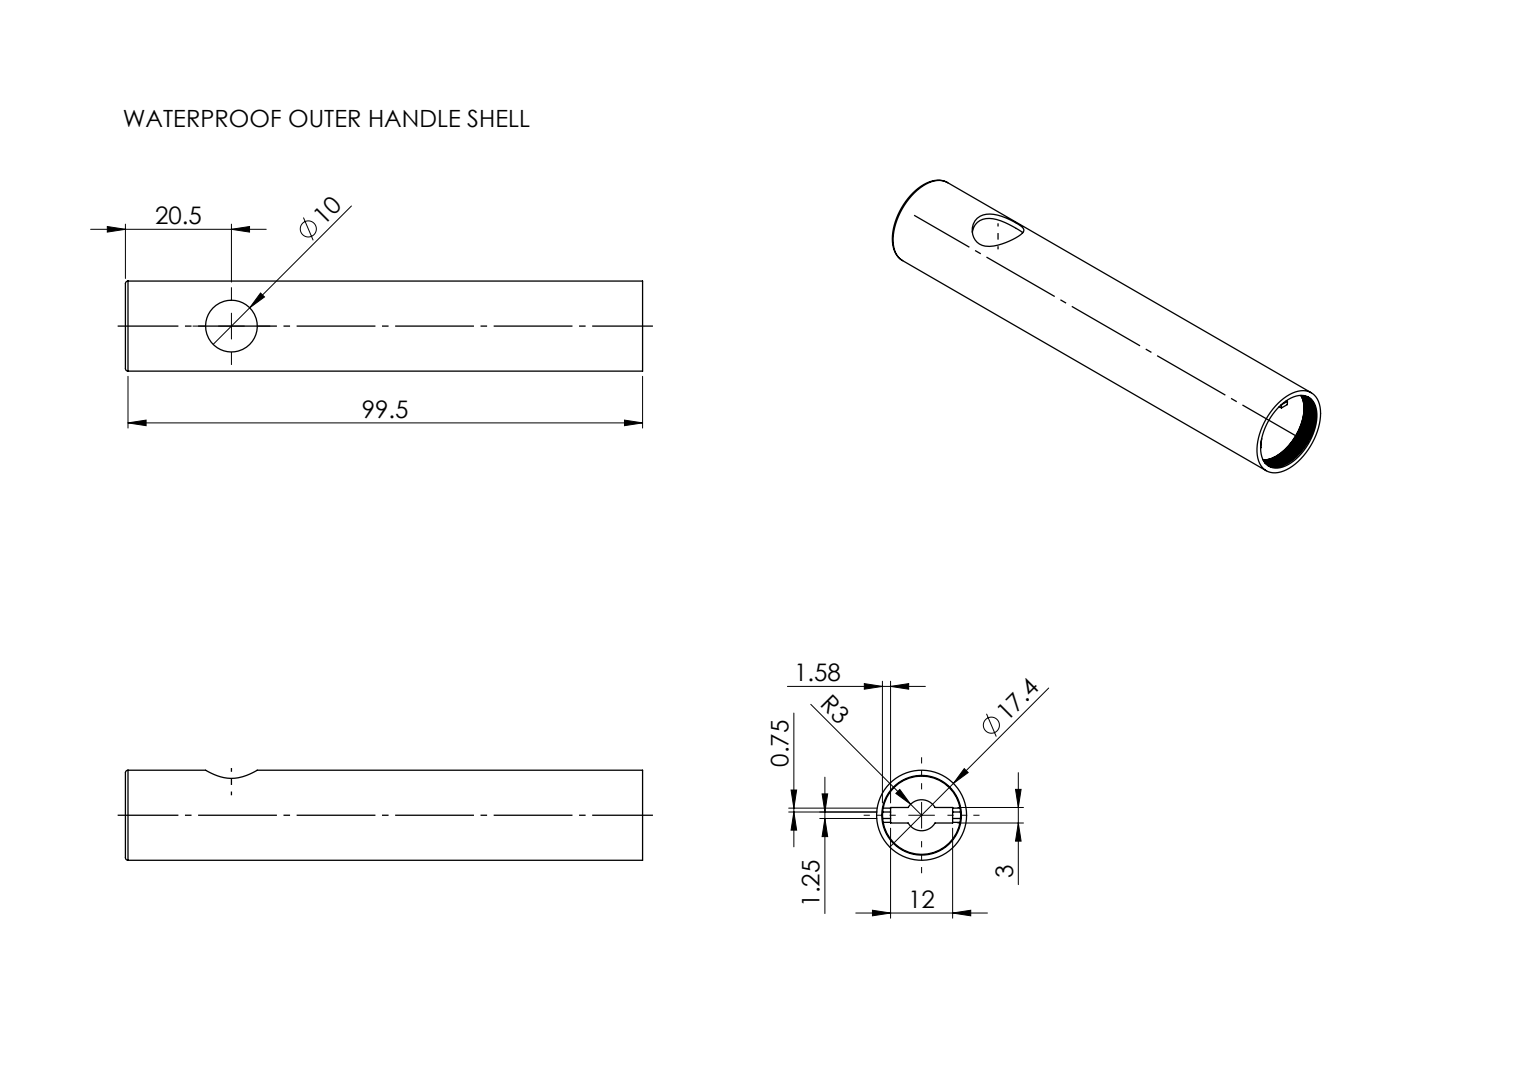
ISO-10303-21;
HEADER;
FILE_DESCRIPTION (('STEP AP214'),
    '1' );
FILE_NAME ('Waterproof Outer Handle Shell.step',
    '2026-10-02T09:26:43',
    ( '' ),
    ( '' ),
    'SwSTEP 2.0',
    'SolidWorks 2026',
    '' );
FILE_SCHEMA (( 'AUTOMOTIVE_DESIGN' ));
ENDSEC;

DATA;
#5=DIRECTION ( 'NONE',  ( -1.000000000000000000, -0.000000000000000000, -0.000000000000000000 ) ) ;
#32=DIRECTION ( 'NONE',  ( 0.000000000000000000, 0.000000000000000000, -1.000000000000000000 ) ) ;
#92=( BOUNDED_CURVE ( )  B_SPLINE_CURVE ( 2, ( #80530, #51076, #39332, #70696, #90980, #28848, #108684 ),
 .UNSPECIFIED., .F., .F. ) 
 B_SPLINE_CURVE_WITH_KNOTS ( ( 3, 2, 2, 3 ),
 ( 0.7142857142857148567, 0.7380952380952386926, 0.7619047619047624176, 0.7857142857142862535 ),
 .UNSPECIFIED. ) 
 CURVE ( )  GEOMETRIC_REPRESENTATION_ITEM ( )  RATIONAL_B_SPLINE_CURVE ( ( 0.9999999999999968914, 0.8660254037844418162, 1.000000000000000000, 0.8660254037844387076, 1.000000000000000000, 0.8660254037844355990, 1.000000000000003109 ) ) 
 REPRESENTATION_ITEM ( '' )  );
#144=CARTESIAN_POINT ( 'NONE',  ( 187.0677083336747160, -4.367472073101514418, -7.564683531250002702 ) ) ;
#216=ORIENTED_EDGE ( 'NONE', *, *, #25647, .T. ) ;
#223=EDGE_CURVE ( 'NONE', #51195, #50358, #69379, .T. ) ;
#245=EDGE_CURVE ( 'NONE', #43167, #39233, #13868, .T. ) ;
#256=CARTESIAN_POINT ( 'NONE',  ( 186.4218750003414016, 0.000000000000000000, 7.564683531250000925 ) ) ;
#346=CARTESIAN_POINT ( 'NONE',  ( 184.9427083336747160, -6.551208109652278289, 3.782341765624995134 ) ) ;
#354=CARTESIAN_POINT ( 'NONE',  ( 185.5000000000000000, 0.000000000000000000, 7.700000000000000178 ) ) ;
#507=CARTESIAN_POINT ( 'NONE',  ( 108.8430433244084554, 5.913955341756470752, 4.931228954127792719 ) ) ;
#548=CARTESIAN_POINT ( 'NONE',  ( 186.6927083336747160, 6.551208109652275624, -3.782341765624998686 ) ) ;
#601=( GEOMETRIC_REPRESENTATION_CONTEXT ( 3 ) GLOBAL_UNCERTAINTY_ASSIGNED_CONTEXT ( ( #63820 ) ) GLOBAL_UNIT_ASSIGNED_CONTEXT ( ( #82675, #124525, #32940 ) ) REPRESENTATION_CONTEXT ( 'NONE', 'WORKASPACE' ) );
#603=EDGE_LOOP ( 'NONE', ( #56647, #48064, #112160, #118008 ) ) ;
#644=CARTESIAN_POINT ( 'NONE',  ( 186.5312500006828031, 9.429780353434619030E-16, -7.700000000000000178 ) ) ;
#695=CARTESIAN_POINT ( 'NONE',  ( 185.9583333333333144, 4.445597072760159030, 7.699999999999928235 ) ) ;
#805=CARTESIAN_POINT ( 'NONE',  ( 103.6746308345937422, 8.329113074144254725, -2.529173134518388544 ) ) ;
#871=( BOUNDED_CURVE ( )  B_SPLINE_CURVE ( 2, ( #122989, #65333, #24143, #44418, #5760, #82436, #64062, #74530, #103993, #54246, #62787, #122352, #72603, #114441, #14300, #84347, #124279, #24787, #64699, #104620, #14922, #13000, #92895, #54872, #98660, #115730, #8351, #126205, #117004, #47654, #97383, #18820, #27336, #35892, #108489, #98027, #46344, #118313, #127501, #26719, #106553, #75801, #26080, #58758, #86258, #87556, #37194, #65989, #16856, #16225, #45722, #48292, #68564, #85630, #37824, #125549, #105924, #58122, #56160, #28661, #36556, #96095, #6393, #56790, #78416, #28006, #76467, #67243, #77727, #116371, #86913, #107199, #77108, #66628, #117642, #96726, #7054, #47014, #67923, #38495, #126857, #17525, #107850, #57473, #7702 ),
 .UNSPECIFIED., .F., .F. ) 
 B_SPLINE_CURVE_WITH_KNOTS ( ( 3, 2, 2, 2, 2, 2, 2, 2, 2, 2, 2, 2, 2, 2, 2, 2, 2, 2, 2, 2, 2, 2, 2, 2, 2, 2, 2, 2, 2, 2, 2, 2, 2, 2, 2, 2, 2, 2, 2, 2, 2, 2, 3 ),
 ( 0.000000000000000000, 0.02380952380952380820, 0.04761904761904761640, 0.07142857142857142461, 0.09523809523809523281, 0.1190476190476190410, 0.1428571428571428492, 0.1666666666666666574, 0.1904761904761904656, 0.2142857142857142738, 0.2380952380952380820, 0.2619047619047619180, 0.2857142857142856984, 0.3095238095238095344, 0.3333333333333333148, 0.3571428571428571508, 0.3809523809523809312, 0.4047619047619047672, 0.4285714285714285476, 0.4523809523809523836, 0.4761904761904761640, 0.5000000000000000000, 0.5238095238095238360, 0.5476190476190476719, 0.5714285714285713969, 0.5952380952380952328, 0.6190476190476190688, 0.6428571428571429047, 0.6666666666666666297, 0.6904761904761904656, 0.7142857142857143016, 0.7380952380952381375, 0.7619047619047618625, 0.7857142857142856984, 0.8095238095238095344, 0.8333333333333333703, 0.8571428571428570953, 0.8809523809523809312, 0.9047619047619047672, 0.9285714285714286031, 0.9523809523809523281, 0.9761904761904761640, 1.000000000000000000 ),
 .UNSPECIFIED. ) 
 CURVE ( )  GEOMETRIC_REPRESENTATION_ITEM ( )  RATIONAL_B_SPLINE_CURVE ( ( 1.000000000000000000, 0.8660254037844387076, 1.000000000000000000, 0.8660254037844387076, 1.000000000000000000, 0.8660254037844387076, 1.000000000000000000, 0.8660254037844387076, 1.000000000000000000, 0.8660254037844387076, 1.000000000000000000, 0.8660254037844387076, 1.000000000000000000, 0.8660254037844387076, 1.000000000000000000, 0.8660254037844387076, 1.000000000000000000, 0.8660254037844387076, 1.000000000000000000, 0.8660254037844387076, 1.000000000000000000, 0.8660254037844387076, 1.000000000000000000, 0.8660254037844387076, 1.000000000000000000, 0.8660254037844387076, 1.000000000000000000, 0.8660254037844387076, 1.000000000000000000, 0.8660254037844387076, 1.000000000000000000, 0.8660254037844387076, 1.000000000000000000, 0.8660254037844387076, 1.000000000000000000, 0.8660254037844387076, 1.000000000000000000, 0.8660254037844387076, 1.000000000000000000, 0.8660254037844387076, 1.000000000000000000, 0.8660254037844387076, 1.000000000000000000, 0.8660254037844387076, 1.000000000000000000, 0.8660254037844387076, 1.000000000000000000, 0.8660254037844387076, 1.000000000000000000, 0.8660254037844387076, 1.000000000000000000, 0.8660254037844387076, 1.000000000000000000, 0.8660254037844387076, 1.000000000000000000, 0.8660254037844387076, 1.000000000000000000, 0.8660254037844387076, 1.000000000000000000, 0.8660254037844387076, 1.000000000000000000, 0.8660254037844387076, 1.000000000000000000, 0.8660254037844387076, 1.000000000000000000, 0.8660254037844387076, 1.000000000000000000, 0.8660254037844387076, 1.000000000000000000, 0.8660254037844387076, 1.000000000000000000, 0.8660254037844387076, 1.000000000000000000, 0.8660254037844387076, 1.000000000000000000, 0.8660254037844387076, 1.000000000000000000, 0.8660254037844387076, 1.000000000000000000, 0.8660254037844387076, 1.000000000000000000, 0.8660254037844387076, 1.000000000000000000, 0.8660254037844387076, 1.000000000000000000 ) ) 
 REPRESENTATION_ITEM ( '' )  );
#888=CARTESIAN_POINT ( 'NONE',  ( 111.9626685488627942, 8.146665828590855085, 3.066327037116900023 ) ) ;
#912=EDGE_CURVE ( 'NONE', #19872, #5682, #21151, .T. ) ;
#921=CARTESIAN_POINT ( 'NONE',  ( 184.2916666666666856, 4.445597072760049784, -7.700000000000123634 ) ) ;
#993=ORIENTED_EDGE ( 'NONE', *, *, #126584, .F. ) ;
#1000=VERTEX_POINT ( 'NONE', #9044 ) ;
#1007=CARTESIAN_POINT ( 'NONE',  ( 183.9843750003414016, -8.734944146203032389, -1.604583208406768146E-15 ) ) ;
#1008=PLANE ( 'NONE',  #81316 ) ;
#1098=ORIENTED_EDGE ( 'NONE', *, *, #72625, .T. ) ;
#1111=AXIS2_PLACEMENT_3D ( 'NONE', #4715, #13259, #63021 ) ;
#1117=CARTESIAN_POINT ( 'NONE',  ( 187.5000000000000000, 0.000000000000000000, 0.000000000000000000 ) ) ;
#1139=DIRECTION ( 'NONE',  ( 0.000000000000000000, 1.000000000000000000, 0.000000000000000000 ) ) ;
#1204=CARTESIAN_POINT ( 'NONE',  ( 184.8593750003413732, 0.000000000000000000, 7.564683531250000925 ) ) ;
#1226=ADVANCED_FACE ( 'NONE', ( #124820 ), #52852, .F. ) ;
#1327=DIRECTION ( 'NONE',  ( -1.000000000000000000, -0.000000000000000000, -0.000000000000000000 ) ) ;
#1392=VERTEX_POINT ( 'NONE', #77482 ) ;
#1410=CARTESIAN_POINT ( 'NONE',  ( 183.8906250003414016, 0.000000000000000000, 7.564683531250000925 ) ) ;
#1445=CARTESIAN_POINT ( 'NONE',  ( 186.1093750003413732, 9.264065473108010111E-16, -7.564683531250000925 ) ) ;
#1551=CARTESIAN_POINT ( 'NONE',  ( 187.1302083336747444, -4.367472073101514418, -7.564683531250002702 ) ) ;
#1629=EDGE_CURVE ( 'NONE', #101564, #44902, #5358, .T. ) ;
#1630=B_SPLINE_CURVE_WITH_KNOTS ( 'NONE', 3,
 ( #25452, #14975, #54922, #124969, #75216, #57521, #49000, #29997, #90167, #9042, #69914, #78465, #28706, #127544, #88911, #98707, #118358, #8396, #60112, #20165, #98075, #88229, #67964, #97429, #107895, #48336, #68611, #7755, #89547, #100021, #10342, #128193, #50275, #507, #108546, #49645, #128861, #129506 ),
 .UNSPECIFIED., .F., .F.,
 ( 4, 2, 2, 2, 2, 2, 2, 2, 2, 2, 2, 2, 2, 2, 2, 2, 2, 2, 4 ),
 ( 0.000000000000000000, 0.001007299096406573174, 0.002014598192813146348, 0.003021897289219719306, 0.004029196385626292697, 0.005036495482032866088, 0.006043794578439438611, 0.007051093674846012002, 0.008058392771252585393, 0.008562042319455872089, 0.009065691867659158784, 0.01007299096406573218, 0.01108029006047230557, 0.01208758915687887722, 0.01309488825328545061, 0.01410218734969202400, 0.01510948644609859740, 0.01561313599430188409, 0.01611678554250517079 ),
 .UNSPECIFIED. ) ;
#1698=EDGE_CURVE ( 'NONE', #109625, #1000, #112399, .T. ) ;
#1819=ADVANCED_FACE ( 'NONE', ( #89728 ), #48520, .F. ) ;
#1840=ORIENTED_EDGE ( 'NONE', *, *, #49030, .T. ) ;
#1841=CARTESIAN_POINT ( 'NONE',  ( 186.2968750003414584, 8.734944146203032389, 5.348610694689227483E-16 ) ) ;
#1861=CYLINDRICAL_SURFACE ( 'NONE', #39546, 7.700000000000000178 ) ;
#1865=CARTESIAN_POINT ( 'NONE',  ( 127.5000000000000000, 0.000000000000000000, 0.000000000000000000 ) ) ;
#1966=ORIENTED_EDGE ( 'NONE', *, *, #68617, .F. ) ;
#1967=CARTESIAN_POINT ( 'NONE',  ( 103.0694403040216400, 7.655046866769239955, 0.8471574321703054800 ) ) ;
#2046=VERTEX_POINT ( 'NONE', #63497 ) ;
#2074=FACE_OUTER_BOUND ( 'NONE', #73731, .T. ) ;
#2081=CARTESIAN_POINT ( 'NONE',  ( 184.7760416670080588, 6.551208109652274736, 3.782341765625001351 ) ) ;
#2171=VERTEX_POINT ( 'NONE', #83148 ) ;
#2265=ORIENTED_EDGE ( 'NONE', *, *, #128795, .F. ) ;
#2305=CARTESIAN_POINT ( 'NONE',  ( 187.5000000000000000, -1.500000000000000000, 6.000000000000000000 ) ) ;
#2347=ORIENTED_EDGE ( 'NONE', *, *, #100683, .T. ) ;
#2370=( BOUNDED_CURVE ( )  B_SPLINE_CURVE ( 2, ( #36862, #103671, #76781, #74847, #23816, #114754, #54535 ),
 .UNSPECIFIED., .F., .F. ) 
 B_SPLINE_CURVE_WITH_KNOTS ( ( 3, 2, 2, 3 ),
 ( 0.2142857142857144681, 0.2380952380952383041, 0.2619047619047621955, 0.2857142857142859760 ),
 .UNSPECIFIED. ) 
 CURVE ( )  GEOMETRIC_REPRESENTATION_ITEM ( )  RATIONAL_B_SPLINE_CURVE ( ( 0.9999999999999988898, 0.8660254037844397068, 1.000000000000000000, 0.8660254037844387076, 1.000000000000000000, 0.8660254037844371533, 1.000000000000001554 ) ) 
 REPRESENTATION_ITEM ( '' )  );
#2428=CARTESIAN_POINT ( 'NONE',  ( 185.9479166673494603, -6.668395609140176816, -3.850000000000003642 ) ) ;
#2475=CARTESIAN_POINT ( 'NONE',  ( 186.3802083336747444, 4.367472073101515306, 7.564683531250000925 ) ) ;
#2523=EDGE_CURVE ( 'NONE', #39233, #127679, #43323, .T. ) ;
#2635=CARTESIAN_POINT ( 'NONE',  ( 186.0312500006828031, 9.429780353434619030E-16, -7.700000000000000178 ) ) ;
#2688=CARTESIAN_POINT ( 'NONE',  ( 108.0000000000000142, 8.700999999999998735, -5.000000000000004441 ) ) ;
#2711=CIRCLE ( 'NONE', #46527, 7.700000000000000178 ) ;
#2729=CARTESIAN_POINT ( 'NONE',  ( 185.2760416670080588, 6.551208109652274736, 3.782341765625001351 ) ) ;
#2798=DIRECTION ( 'NONE',  ( -1.000000000000000000, -0.000000000000000000, -0.000000000000000000 ) ) ;
#2847=CARTESIAN_POINT ( 'NONE',  ( 185.6718750003414016, 9.264065473108010111E-16, -7.564683531250000925 ) ) ;
#2865=VECTOR ( 'NONE', #65208, 1000.000000000000000 ) ;
#2879=CARTESIAN_POINT ( 'NONE',  ( 129.5000000000000000, 0.6250000000000025535, -6.000000000000000888 ) ) ;
#2922=CARTESIAN_POINT ( 'NONE',  ( 127.5000000000000000, 0.000000000000000000, 0.000000000000000000 ) ) ;
#2955=CARTESIAN_POINT ( 'NONE',  ( 187.5000000000000000, 9.429780353434619030E-16, -7.700000000000000178 ) ) ;
#2977=PLANE ( 'NONE',  #102632 ) ;
#3027=CARTESIAN_POINT ( 'NONE',  ( 187.5000000000000000, 0.000000000000000000, 0.000000000000000000 ) ) ;
#3105=CARTESIAN_POINT ( 'NONE',  ( 186.1145833340161175, 6.668395609140177704, -3.849999999999998312 ) ) ;
#3151=CARTESIAN_POINT ( 'NONE',  ( 186.3385416670080872, 6.551208109652274736, 3.782341765625001351 ) ) ;
#3193=EDGE_CURVE ( 'NONE', #125237, #48297, #19068, .T. ) ;
#3379=DIRECTION ( 'NONE',  ( 0.000000000000000000, 0.000000000000000000, -1.000000000000000000 ) ) ;
#3381=CARTESIAN_POINT ( 'NONE',  ( 184.4843750003414016, -8.734944146203032389, -1.604583208406767949E-15 ) ) ;
#3422=ORIENTED_EDGE ( 'NONE', *, *, #86612, .T. ) ;
#3426=ORIENTED_EDGE ( 'NONE', *, *, #115420, .F. ) ;
#3452=PRESENTATION_STYLE_ASSIGNMENT (( #104230 ) ) ;
#3495=CARTESIAN_POINT ( 'NONE',  ( 185.5052083336747444, -6.551208109652278289, 3.782341765624995134 ) ) ;
#3521=DIRECTION ( 'NONE',  ( 1.000000000000000000, 0.000000000000000000, 0.000000000000000000 ) ) ;
#3526=ORIENTED_EDGE ( 'NONE', *, *, #20363, .F. ) ;
#3554=LINE ( 'NONE', #4823, #108100 ) ;
#3588=AXIS2_PLACEMENT_3D ( 'NONE', #42405, #90849, #92793 ) ;
#3675=CARTESIAN_POINT ( 'NONE',  ( 179.5000000000000000, 0.6250000000000000000, 7.634788798650556707 ) ) ;
#3732=CARTESIAN_POINT ( 'NONE',  ( 187.2812500006828031, 0.000000000000000000, 7.700000000000000178 ) ) ;
#3736=ORIENTED_EDGE ( 'NONE', *, *, #125313, .T. ) ;
#3786=CARTESIAN_POINT ( 'NONE',  ( 186.0052083336747444, -6.551208109652278289, 3.782341765624995134 ) ) ;
#3815=CYLINDRICAL_SURFACE ( 'NONE', #8172, 7.700000000000000178 ) ;
#3837=VERTEX_POINT ( 'NONE', #33900 ) ;
#3844=VECTOR ( 'NONE', #11494, 1000.000000000000000 ) ;
#3915=LINE ( 'NONE', #83769, #106167 ) ;
#3962=CARTESIAN_POINT ( 'NONE',  ( 179.5000000000000000, 0.9999999999999985567, -7.634788798650556707 ) ) ;
#3991=CARTESIAN_POINT ( 'NONE',  ( 179.5000000000000000, 0.6250000000000000000, 7.634788798650556707 ) ) ;
#4018=CARTESIAN_POINT ( 'NONE',  ( 186.3593750003414016, 0.000000000000000000, 7.564683531250000925 ) ) ;
#4038=DIRECTION ( 'NONE',  ( 0.4999999999999471534, 0.000000000000000000, 0.8660254037844692387 ) ) ;
#4119=CARTESIAN_POINT ( 'NONE',  ( 184.5885416670080872, -6.551208109652273848, -3.782341765625003571 ) ) ;
#4120=LINE ( 'NONE', #104275, #101288 ) ;
#4350=CARTESIAN_POINT ( 'NONE',  ( 186.2395833340161460, 4.445597072760117285, 7.699999999999999289 ) ) ;
#4393=CARTESIAN_POINT ( 'NONE',  ( 184.4218750003414016, 0.000000000000000000, 7.564683531250000925 ) ) ;
#4404=DIRECTION ( 'NONE',  ( 0.000000000000000000, 0.000000000000000000, 1.000000000000000000 ) ) ;
#4435=VERTEX_POINT ( 'NONE', #79673 ) ;
#4467=EDGE_CURVE ( 'NONE', #69479, #8359, #49593, .T. ) ;
#4600=EDGE_LOOP ( 'NONE', ( #92441, #71078, #11723, #98558, #76871, #216, #64515, #90448, #67535, #43861, #22545, #129524 ) ) ;
#4602=DIRECTION ( 'NONE',  ( 0.000000000000000000, -1.000000000000000000, 0.000000000000000000 ) ) ;
#4715=CARTESIAN_POINT ( 'NONE',  ( 88.00000000000001421, 0.000000000000000000, 0.000000000000000000 ) ) ;
#4736=VERTEX_POINT ( 'NONE', #95299 ) ;
#4759=CARTESIAN_POINT ( 'NONE',  ( 185.9218750003414016, 0.000000000000000000, 7.564683531250000925 ) ) ;
#4823=CARTESIAN_POINT ( 'NONE',  ( 129.5000000000000000, 0.000000000000000000, -6.000000000000000000 ) ) ;
#4965=DIRECTION ( 'NONE',  ( -1.000000000000000000, -0.000000000000000000, -0.000000000000000000 ) ) ;
#4989=ORIENTED_EDGE ( 'NONE', *, *, #39742, .T. ) ;
#5012=CARTESIAN_POINT ( 'NONE',  ( 186.9427083336747160, -6.551208109652278289, 3.782341765624995134 ) ) ;
#5017=EDGE_LOOP ( 'NONE', ( #24373, #85596, #89158, #101784, #111936 ) ) ;
#5054=LINE ( 'NONE', #124847, #24714 ) ;
#5058=SHAPE_REPRESENTATION ( 'Waterproof Outer Handle Shell', ( #108296 ), #20574 ) ;
#5061=CARTESIAN_POINT ( 'NONE',  ( 185.7552083336747444, 6.551208109652275624, -3.782341765624998686 ) ) ;
#5158=DIRECTION ( 'NONE',  ( 1.000000000000000000, 0.000000000000000000, 0.000000000000000000 ) ) ;
#5250=VERTEX_POINT ( 'NONE', #14619 ) ;
#5260=DIRECTION ( 'NONE',  ( 0.000000000000000000, 0.000000000000000000, 1.000000000000000000 ) ) ;
#5358=LINE ( 'NONE', #115290, #64269 ) ;
#5416=CARTESIAN_POINT ( 'NONE',  ( 184.2968750003414300, 8.734944146203032389, 5.348610694689227483E-16 ) ) ;
#5448=AXIS2_PLACEMENT_3D ( 'NONE', #6276, #103213, #13531 ) ;
#5608=PLANE ( 'NONE',  #75805 ) ;
#5616=ORIENTED_EDGE ( 'NONE', *, *, #14550, .T. ) ;
#5652=CARTESIAN_POINT ( 'NONE',  ( 186.8593750003414016, 0.000000000000000000, 7.564683531250000925 ) ) ;
#5682=VERTEX_POINT ( 'NONE', #60243 ) ;
#5699=CARTESIAN_POINT ( 'NONE',  ( 184.6718750003414016, 9.264065473108010111E-16, -7.564683531250000925 ) ) ;
#5760=CARTESIAN_POINT ( 'NONE',  ( 187.2552083336747444, 6.551208109652275624, -3.782341765624998686 ) ) ;
#5891=DIRECTION ( 'NONE',  ( 0.000000000000000000, 0.000000000000000000, -1.000000000000000000 ) ) ;
#6053=CARTESIAN_POINT ( 'NONE',  ( 186.2916666666666856, 4.445597072760120838, -7.699999999999998401 ) ) ;
#6152=ORIENTED_EDGE ( 'NONE', *, *, #63330, .T. ) ;
#6158=CARTESIAN_POINT ( 'NONE',  ( 179.5000000000000000, 0.000000000000000000, 0.000000000000000000 ) ) ;
#6176=EDGE_LOOP ( 'NONE', ( #25164, #59153, #99939, #22610 ) ) ;
#6275=ORIENTED_EDGE ( 'NONE', *, *, #58862, .T. ) ;
#6276=CARTESIAN_POINT ( 'NONE',  ( 88.00000000000001421, 0.000000000000000000, 0.000000000000000000 ) ) ;
#6289=CARTESIAN_POINT ( 'NONE',  ( 185.1562500006828031, 8.891194145520236347, 5.444286225454521982E-16 ) ) ;
#6327=CARTESIAN_POINT ( 'NONE',  ( 185.6302083336747444, -4.367472073101514418, -7.564683531250002702 ) ) ;
#6393=CARTESIAN_POINT ( 'NONE',  ( 184.8385416670080872, 6.551208109652274736, 3.782341765625001351 ) ) ;
#6439=CARTESIAN_POINT ( 'NONE',  ( 87.50000000000001421, 0.000000000000000000, 0.000000000000000000 ) ) ;
#6544=FACE_BOUND ( 'NONE', #57159, .T. ) ;
#6621=AXIS2_PLACEMENT_3D ( 'NONE', #55391, #126049, #114937 ) ;
#6678=EDGE_CURVE ( 'NONE', #126401, #27968, #86827, .T. ) ;
#6680=CARTESIAN_POINT ( 'NONE',  ( 186.1250000000000000, -8.891194145520236347, -1.633285867636356693E-15 ) ) ;
#6760=EDGE_LOOP ( 'NONE', ( #22469, #86308, #59191, #98544 ) ) ;
#6784=CARTESIAN_POINT ( 'NONE',  ( 184.7500000000000000, 9.429780353434619030E-16, -7.700000000000000178 ) ) ;
#6793=VECTOR ( 'NONE', #72656, 1000.000000000000000 ) ;
#6801=CARTESIAN_POINT ( 'NONE',  ( 186.2500000000000000, 9.429780353434619030E-16, -7.700000000000000178 ) ) ;
#6916=ORIENTED_EDGE ( 'NONE', *, *, #50030, .F. ) ;
#6928=CARTESIAN_POINT ( 'NONE',  ( 187.1510416670080303, 4.367472073101518859, -7.564683531249999149 ) ) ;
#6974=CARTESIAN_POINT ( 'NONE',  ( 184.5885416670080872, -6.551208109652273848, -3.782341765625003571 ) ) ;
#6995=VECTOR ( 'NONE', #108172, 1000.000000000000000 ) ;
#7054=CARTESIAN_POINT ( 'NONE',  ( 184.2552083336747444, 6.551208109652275624, -3.782341765624998686 ) ) ;
#7161=EDGE_LOOP ( 'NONE', ( #21529, #9268, #66233, #100365 ) ) ;
#7166=EDGE_CURVE ( 'NONE', #27968, #129597, #16895, .T. ) ;
#7174=AXIS2_PLACEMENT_3D ( 'NONE', #78334, #68486, #108408 ) ;
#7236=CARTESIAN_POINT ( 'NONE',  ( 185.6145833340161175, 6.668395609140177704, -3.849999999999998312 ) ) ;
#7344=CARTESIAN_POINT ( 'NONE',  ( 184.9583333333333144, 4.445597072760117285, 7.699999999999999289 ) ) ;
#7348=CYLINDRICAL_SURFACE ( 'NONE', #103980, 7.700000000000000178 ) ;
#7411=VECTOR ( 'NONE', #60214, 1000.000000000000000 ) ;
#7448=CIRCLE ( 'NONE', #124544, 7.700000000000000178 ) ;
#7596=CARTESIAN_POINT ( 'NONE',  ( 187.0260416670080588, -6.551208109652273848, -3.782341765625003571 ) ) ;
#7606=VERTEX_POINT ( 'NONE', #95349 ) ;
#7620=LINE ( 'NONE', #66543, #53358 ) ;
#7702=CARTESIAN_POINT ( 'NONE',  ( 183.9218750003414016, 0.000000000000000000, 7.564683531250000925 ) ) ;
#7755=CARTESIAN_POINT ( 'NONE',  ( 111.3044611531193766, 6.721044513813564159, 3.765782231328828722 ) ) ;
#7931=FILL_AREA_STYLE ('',( #98896 ) ) ;
#7959=AXIS2_PLACEMENT_3D ( 'NONE', #15797, #38025, #88395 ) ;
#7994=CARTESIAN_POINT ( 'NONE',  ( 186.3333333333333144, 6.668395609140177704, -3.849999999999998312 ) ) ;
#8037=EDGE_CURVE ( 'NONE', #77053, #99802, #75202, .T. ) ;
#8039=CARTESIAN_POINT ( 'NONE',  ( 187.3177083336747160, 4.367472073101515306, 7.564683531250000925 ) ) ;
#8159=EDGE_CURVE ( 'NONE', #79874, #74365, #18850, .T. ) ;
#8168=DIRECTION ( 'NONE',  ( 0.000000000000000000, 0.000000000000000000, 1.000000000000000000 ) ) ;
#8172=AXIS2_PLACEMENT_3D ( 'NONE', #32664, #102652, #13623 ) ;
#8177=DIRECTION ( 'NONE',  ( 1.000000000000000000, 0.000000000000000000, 0.000000000000000000 ) ) ;
#8196=CARTESIAN_POINT ( 'NONE',  ( 184.8750000000000000, 8.891194145520236347, 5.444286225454521982E-16 ) ) ;
#8285=AXIS2_PLACEMENT_3D ( 'NONE', #49276, #21738, #99001 ) ;
#8351=CARTESIAN_POINT ( 'NONE',  ( 186.3385416670080872, 6.551208109652274736, 3.782341765625001351 ) ) ;
#8359=VERTEX_POINT ( 'NONE', #110456 ) ;
#8369=FACE_OUTER_BOUND ( 'NONE', #12876, .T. ) ;
#8396=CARTESIAN_POINT ( 'NONE',  ( 113.0003993415903523, 7.700259312267349721, 0.1577655332996449056 ) ) ;
#8404=ORIENTED_EDGE ( 'NONE', *, *, #40841, .T. ) ;
#8432=CARTESIAN_POINT ( 'NONE',  ( 186.5677083336747160, -4.367472073101514418, -7.564683531250002702 ) ) ;
#8505=ORIENTED_EDGE ( 'NONE', *, *, #106734, .F. ) ;
#8566=CARTESIAN_POINT ( 'NONE',  ( 185.8750000000000000, 8.891194145520236347, 5.444286225454521982E-16 ) ) ;
#8625=CARTESIAN_POINT ( 'NONE',  ( 184.5416666666666572, -4.445597072760122614, 7.699999999999998401 ) ) ;
#8660=ADVANCED_FACE ( 'NONE', ( #42229 ), #62520, .T. ) ;
#8670=CARTESIAN_POINT ( 'NONE',  ( 107.3283734746308227, 7.144069872249539266, 4.965747202897751400 ) ) ;
#8735=AXIS2_PLACEMENT_3D ( 'NONE', #15402, #105074, #94616 ) ;
#8750=CARTESIAN_POINT ( 'NONE',  ( 111.3045913714602477, 7.846616099438112890, 3.765819408771217347 ) ) ;
#8875=CARTESIAN_POINT ( 'NONE',  ( 185.1510416670080872, 4.367472073101518859, -7.564683531249999149 ) ) ;
#8955=EDGE_LOOP ( 'NONE', ( #49758, #116316, #27736, #11281 ) ) ;
#9042=CARTESIAN_POINT ( 'NONE',  ( 111.7496660746278820, 6.950752061642088364, -3.322700296524552233 ) ) ;
#9044=CARTESIAN_POINT ( 'NONE',  ( 87.50000000000001421, 0.000000000000000000, -8.199999999999999289 ) ) ;
#9087=ORIENTED_EDGE ( 'NONE', *, *, #82659, .F. ) ;
#9089=CARTESIAN_POINT ( 'NONE',  ( 186.1927083336747160, 6.551208109652275624, -3.782341765624998686 ) ) ;
#9226=CARTESIAN_POINT ( 'NONE',  ( 107.9999999999992895, 5.855766388783293586, 5.000000000000080824 ) ) ;
#9238=SURFACE_SIDE_STYLE ('',( #47882 ) ) ;
#9268=ORIENTED_EDGE ( 'NONE', *, *, #112266, .T. ) ;
#9278=ORIENTED_EDGE ( 'NONE', *, *, #116510, .F. ) ;
#9338=CARTESIAN_POINT ( 'NONE',  ( 186.6510416670080872, 4.367472073101518859, -7.564683531249999149 ) ) ;
#9343=CARTESIAN_POINT ( 'NONE',  ( 103.5197895262259493, 8.411351917275529999, -2.243970670365522224 ) ) ;
#9389=CARTESIAN_POINT ( 'NONE',  ( 185.0000000000000000, 0.000000000000000000, 7.700000000000000178 ) ) ;
#9422=CARTESIAN_POINT ( 'NONE',  ( 112.4803320538941875, 8.411414713183589242, 2.243816228936815538 ) ) ;
#9429=EDGE_CURVE ( 'NONE', #69132, #114300, #128120, .T. ) ;
#9548=CARTESIAN_POINT ( 'NONE',  ( 186.2760416670080588, 6.551208109652274736, 3.782341765625001351 ) ) ;
#9718=ORIENTED_EDGE ( 'NONE', *, *, #42804, .T. ) ;
#9730=CARTESIAN_POINT ( 'NONE',  ( 185.7083333333333428, -4.445597072760163471, -7.699999999999919353 ) ) ;
#9738=VERTEX_POINT ( 'NONE', #92119 ) ;
#9739=CARTESIAN_POINT ( 'NONE',  ( 185.6510416670080303, 4.367472073101518859, -7.564683531249999149 ) ) ;
#9766=CARTESIAN_POINT ( 'NONE',  ( 129.5000000000000000, 0.000000000000000000, -6.000000000000000000 ) ) ;
#9799=CARTESIAN_POINT ( 'NONE',  ( 184.5312500006828031, 9.429780353434619030E-16, -7.700000000000000178 ) ) ;
#9871=CARTESIAN_POINT ( 'NONE',  ( 104.7003906511443461, 6.718614722302491238, 3.770225884972850494 ) ) ;
#9878=DIRECTION ( 'NONE',  ( 0.000000000000000000, -1.846105847067148515E-16, -1.000000000000000000 ) ) ;
#9907=ORIENTED_EDGE ( 'NONE', *, *, #115339, .T. ) ;
#9985=CARTESIAN_POINT ( 'NONE',  ( 187.1093750003414016, 9.264065473108010111E-16, -7.564683531250000925 ) ) ;
#9988=CARTESIAN_POINT ( 'NONE',  ( 129.5000000000000000, 1.500000000000000000, 6.000000000000000000 ) ) ;
#9989=CARTESIAN_POINT ( 'NONE',  ( 103.1666495638042278, 8.605133039442083742, 1.322232749994941781 ) ) ;
#10065=CARTESIAN_POINT ( 'NONE',  ( 109.7910216395279122, 7.340097168400048666, 4.671023614519715927 ) ) ;
#10093=CARTESIAN_POINT ( 'NONE',  ( 186.6718750003414016, 9.264065473108010111E-16, -7.564683531250000925 ) ) ;
#10102=DIRECTION ( 'NONE',  ( 0.000000000000000000, -1.846105847067148022E-16, 1.000000000000000000 ) ) ;
#10128=VECTOR ( 'NONE', #67257, 1000.000000000000000 ) ;
#10152=VECTOR ( 'NONE', #103447, 1000.000000000000000 ) ;
#10189=CARTESIAN_POINT ( 'NONE',  ( 185.7343750003414016, 8.734944146203032389, 5.348610694689227483E-16 ) ) ;
#10204=EDGE_CURVE ( 'NONE', #93739, #121068, #124363, .T. ) ;
#10269=EDGE_CURVE ( 'NONE', #13525, #68129, #85961, .T. ) ;
#10329=DIRECTION ( 'NONE',  ( 1.000000000000000000, 0.000000000000000000, 0.000000000000000000 ) ) ;
#10342=CARTESIAN_POINT ( 'NONE',  ( 110.2489501364907198, 6.266397739826595092, 4.477399565010155236 ) ) ;
#10382=CARTESIAN_POINT ( 'NONE',  ( 185.2343750003414016, 8.734944146203032389, 5.348610694689227483E-16 ) ) ;
#10404=CARTESIAN_POINT ( 'NONE',  ( 186.2395833340161175, 4.445597072760147483, 7.699999999999948663 ) ) ;
#10414=ORIENTED_EDGE ( 'NONE', *, *, #14397, .F. ) ;
#10456=DIRECTION ( 'NONE',  ( 0.000000000000000000, -1.000000000000000000, 0.000000000000000000 ) ) ;
#10467=DIRECTION ( 'NONE',  ( 0.000000000000000000, 0.000000000000000000, 1.000000000000000000 ) ) ;
#10538=ORIENTED_EDGE ( 'NONE', *, *, #25647, .F. ) ;
#10553=EDGE_CURVE ( 'NONE', #128041, #16283, #63010, .T. ) ;
#10603=EDGE_CURVE ( 'NONE', #94142, #57508, #45992, .T. ) ;
#10644=CARTESIAN_POINT ( 'NONE',  ( 0.000000000000000000, 0.000000000000000000, 0.000000000000000000 ) ) ;
#10707=CARTESIAN_POINT ( 'NONE',  ( 186.0885416670080872, -6.551208109652273848, -3.782341765625003571 ) ) ;
#10712=CARTESIAN_POINT ( 'NONE',  ( 179.5000000000000000, 0.000000000000000000, 0.000000000000000000 ) ) ;
#10728=CARTESIAN_POINT ( 'NONE',  ( 187.3593750003414016, 0.000000000000000000, 7.564683531250000925 ) ) ;
#10795=CARTESIAN_POINT ( 'NONE',  ( 185.8177083336747444, 4.367472073101515306, 7.564683531250000925 ) ) ;
#10812=DIRECTION ( 'NONE',  ( -1.000000000000000000, -0.000000000000000000, -0.000000000000000000 ) ) ;
#10845=CARTESIAN_POINT ( 'NONE',  ( 179.5000000000000000, -1.000000000000025535, 7.634788798650553154 ) ) ;
#11008=CARTESIAN_POINT ( 'NONE',  ( 185.0677083336747160, -4.367472073101514418, -7.564683531250002702 ) ) ;
#11235=ORIENTED_EDGE ( 'NONE', *, *, #81186, .T. ) ;
#11245=EDGE_CURVE ( 'NONE', #65955, #103176, #16933, .T. ) ;
#11246=ORIENTED_EDGE ( 'NONE', *, *, #86637, .T. ) ;
#11263=CARTESIAN_POINT ( 'NONE',  ( 185.4427083336747160, -6.551208109652278289, 3.782341765624995134 ) ) ;
#11281=ORIENTED_EDGE ( 'NONE', *, *, #113984, .F. ) ;
#11308=EDGE_CURVE ( 'NONE', #5250, #9738, #87636, .T. ) ;
#11375=CARTESIAN_POINT ( 'NONE',  ( 186.5052083336747444, -6.551208109652278289, 3.782341765624995134 ) ) ;
#11380=ORIENTED_EDGE ( 'NONE', *, *, #21604, .T. ) ;
#11381=CARTESIAN_POINT ( 'NONE',  ( 184.2500000000000000, 9.429780353434619030E-16, -7.700000000000000178 ) ) ;
#11412=CARTESIAN_POINT ( 'NONE',  ( 183.9895833340160607, -4.445597072760187451, -7.699999999999876721 ) ) ;
#11448=AXIS2_PLACEMENT_3D ( 'NONE', #47840, #49135, #10467 ) ;
#11494=DIRECTION ( 'NONE',  ( 0.000000000000000000, -0.000000000000000000, -1.000000000000000000 ) ) ;
#11594=ORIENTED_EDGE ( 'NONE', *, *, #13690, .F. ) ;
#11667=CARTESIAN_POINT ( 'NONE',  ( 187.3385416670080872, 6.551208109652274736, 3.782341765625001351 ) ) ;
#11683=EDGE_LOOP ( 'NONE', ( #110846, #107101 ) ) ;
#11713=ORIENTED_EDGE ( 'NONE', *, *, #34242, .F. ) ;
#11723=ORIENTED_EDGE ( 'NONE', *, *, #8159, .F. ) ;
#11758=EDGE_LOOP ( 'NONE', ( #121048, #75033, #84519, #81080, #106240, #113742, #89082, #11246, #100895, #84403, #75375, #87595 ) ) ;
#11818=CYLINDRICAL_SURFACE ( 'NONE', #110333, 7.700000000000000178 ) ;
#11847=CARTESIAN_POINT ( 'NONE',  ( 187.2395833340161460, 4.445597072760117285, 7.700000000000001066 ) ) ;
#11910=CARTESIAN_POINT ( 'NONE',  ( 185.7343750003414016, 8.734944146203032389, 5.348610694689227483E-16 ) ) ;
#11968=CARTESIAN_POINT ( 'NONE',  ( 185.1979166673494603, 6.668395609140176816, 3.850000000000000977 ) ) ;
#12118=DIRECTION ( 'NONE',  ( 0.000000000000000000, 1.846105847067148022E-16, -1.000000000000000000 ) ) ;
#12255=CARTESIAN_POINT ( 'NONE',  ( 186.9062500006828316, -8.891194145520236347, -1.633285867636356693E-15 ) ) ;
#12306=CARTESIAN_POINT ( 'NONE',  ( 184.0677083336747160, -4.367472073101514418, -7.564683531250002702 ) ) ;
#12329=DIRECTION ( 'NONE',  ( -1.000000000000000000, -0.000000000000000000, -0.000000000000000000 ) ) ;
#12431=CARTESIAN_POINT ( 'NONE',  ( 103.2703165085177659, 7.526592624639811824, 1.654927987503729492 ) ) ;
#12495=CARTESIAN_POINT ( 'NONE',  ( 187.2812500006828031, 0.000000000000000000, 7.700000000000000178 ) ) ;
#12547=CARTESIAN_POINT ( 'NONE',  ( 185.6927083336747160, 6.551208109652275624, -3.782341765624998686 ) ) ;
#12583=VERTEX_POINT ( 'NONE', #105061 ) ;
#12637=ORIENTED_EDGE ( 'NONE', *, *, #74034, .F. ) ;
#12640=CARTESIAN_POINT ( 'NONE',  ( 129.5000000000000000, 0.000000000000000000, 0.000000000000000000 ) ) ;
#12647=PLANE ( 'NONE',  #82087 ) ;
#12651=CARTESIAN_POINT ( 'NONE',  ( 187.3385416670080872, 6.551208109652274736, 3.782341765625001351 ) ) ;
#12682=ORIENTED_EDGE ( 'NONE', *, *, #72496, .F. ) ;
#12714=EDGE_LOOP ( 'NONE', ( #85743, #107287 ) ) ;
#12733=ORIENTED_EDGE ( 'NONE', *, *, #63430, .F. ) ;
#12801=LINE ( 'NONE', #113603, #67273 ) ;
#12857=EDGE_LOOP ( 'NONE', ( #80320, #42275, #67492, #84474 ) ) ;
#12876=EDGE_LOOP ( 'NONE', ( #64429, #108536, #82258, #95703 ) ) ;
#12887=CARTESIAN_POINT ( 'NONE',  ( 186.7812500006828031, 0.000000000000000000, 7.700000000000000178 ) ) ;
#12913=EDGE_CURVE ( 'NONE', #73015, #83312, #118675, .T. ) ;
#12938=CARTESIAN_POINT ( 'NONE',  ( 184.1927083336747160, 6.551208109652275624, -3.782341765624998686 ) ) ;
#12958=FACE_OUTER_BOUND ( 'NONE', #29330, .T. ) ;
#12991=ORIENTED_EDGE ( 'NONE', *, *, #18769, .F. ) ;
#13000=CARTESIAN_POINT ( 'NONE',  ( 186.5468750003414300, -8.734944146203032389, -1.604583208406767949E-15 ) ) ;
#13112=MECHANICAL_DESIGN_GEOMETRIC_PRESENTATION_REPRESENTATION('',(#48647),#601);
#13139=ADVANCED_FACE ( 'NONE', ( #77401 ), #69495, .F. ) ;
#13228=ORIENTED_EDGE ( 'NONE', *, *, #86637, .F. ) ;
#13232=LINE ( 'NONE', #23725, #48039 ) ;
#13251=PLANE ( 'NONE',  #86273 ) ;
#13259=DIRECTION ( 'NONE',  ( 1.000000000000000000, 0.000000000000000000, 0.000000000000000000 ) ) ;
#13296=CARTESIAN_POINT ( 'NONE',  ( 187.2500000000000000, 9.429780353434619030E-16, -7.700000000000000178 ) ) ;
#13422=DIRECTION ( 'NONE',  ( 0.000000000000000000, -0.000000000000000000, 1.000000000000000000 ) ) ;
#13433=ORIENTED_EDGE ( 'NONE', *, *, #111619, .T. ) ;
#13469=ORIENTED_EDGE ( 'NONE', *, *, #23025, .T. ) ;
#13477=VECTOR ( 'NONE', #24146, 1000.000000000000000 ) ;
#13507=CARTESIAN_POINT ( 'NONE',  ( 129.5000000000000000, 1.500000000000000000, 2.598076211353316900 ) ) ;
#13525=VERTEX_POINT ( 'NONE', #68060 ) ;
#13531=DIRECTION ( 'NONE',  ( 0.000000000000000000, 0.000000000000000000, -1.000000000000000000 ) ) ;
#13547=CARTESIAN_POINT ( 'NONE',  ( 186.3645833340161175, -6.668395609140180369, 3.849999999999994760 ) ) ;
#13588=CARTESIAN_POINT ( 'NONE',  ( 184.7760416670080588, 6.551208109652274736, 3.782341765625001351 ) ) ;
#13600=CARTESIAN_POINT ( 'NONE',  ( 186.5000000000000000, 0.000000000000000000, 7.700000000000000178 ) ) ;
#13623=DIRECTION ( 'NONE',  ( 0.000000000000000000, 0.000000000000000000, 1.000000000000000000 ) ) ;
#13690=EDGE_CURVE ( 'NONE', #27968, #75118, #104460, .T. ) ;
#13713=EDGE_CURVE ( 'NONE', #18092, #122603, #91765, .T. ) ;
#13720=ORIENTED_EDGE ( 'NONE', *, *, #56646, .F. ) ;
#13729=CARTESIAN_POINT ( 'NONE',  ( 184.9062500006828031, -8.891194145520236347, -1.633285867636356299E-15 ) ) ;
#13746=CARTESIAN_POINT ( 'NONE',  ( 185.8229166673494319, -4.445597072760079982, 7.700000000000070344 ) ) ;
#13761=EDGE_CURVE ( 'NONE', #62383, #61737, #22691, .T. ) ;
#13817=LINE ( 'NONE', #113968, #28508 ) ;
#13834=VECTOR ( 'NONE', #120928, 1000.000000000000000 ) ;
#13837=CARTESIAN_POINT ( 'NONE',  ( 184.8593750003413732, 0.000000000000000000, 7.564683531250000925 ) ) ;
#13868=LINE ( 'NONE', #33535, #104875 ) ;
#13887=DIRECTION ( 'NONE',  ( 0.000000000000000000, 0.000000000000000000, -1.000000000000000000 ) ) ;
#13946=CARTESIAN_POINT ( 'NONE',  ( 184.2552083336747444, 6.551208109652275624, -3.782341765624998686 ) ) ;
#13984=LINE ( 'NONE', #112208, #81585 ) ;
#14183=CARTESIAN_POINT ( 'NONE',  ( 185.4479166673494603, -6.668395609140176816, -3.850000000000003642 ) ) ;
#14214=CARTESIAN_POINT ( 'NONE',  ( 179.5000000000000000, -0.6250000000000000000, 7.634788798650553154 ) ) ;
#14215=DIRECTION ( 'NONE',  ( -1.000000000000000000, -0.000000000000000000, -0.000000000000000000 ) ) ;
#14228=ORIENTED_EDGE ( 'NONE', *, *, #9429, .F. ) ;
#14232=CARTESIAN_POINT ( 'NONE',  ( 184.9427083336747160, -6.551208109652278289, 3.782341765624995134 ) ) ;
#14268=EDGE_LOOP ( 'NONE', ( #53727, #1840, #38894, #46116 ) ) ;
#14300=CARTESIAN_POINT ( 'NONE',  ( 186.8385416670080872, 6.551208109652274736, 3.782341765625001351 ) ) ;
#14397=EDGE_CURVE ( 'NONE', #118850, #50117, #2370, .T. ) ;
#14550=EDGE_CURVE ( 'NONE', #128041, #94142, #19995, .T. ) ;
#14584=CARTESIAN_POINT ( 'NONE',  ( 184.4218750003414016, 0.000000000000000000, 7.564683531250000925 ) ) ;
#14619=CARTESIAN_POINT ( 'NONE',  ( 129.5000000000000000, -0.6250000000000004441, 6.000000000000000000 ) ) ;
#14725=ORIENTED_EDGE ( 'NONE', *, *, #112539, .T. ) ;
#14729=EDGE_CURVE ( 'NONE', #114625, #3837, #13817, .T. ) ;
#14770=CARTESIAN_POINT ( 'NONE',  ( 179.5000000000000000, -1.375000000000000000, 7.634788798650553154 ) ) ;
#14815=CARTESIAN_POINT ( 'NONE',  ( 185.2395833340161175, 4.445597072760117285, 7.699999999999999289 ) ) ;
#14854=DIRECTION ( 'NONE',  ( 0.000000000000000000, 1.000000000000000000, 0.000000000000000000 ) ) ;
#14858=CARTESIAN_POINT ( 'NONE',  ( 185.7135416670080588, 4.367472073101518859, -7.564683531249999149 ) ) ;
#14892=VERTEX_POINT ( 'NONE', #48445 ) ;
#14914=ADVANCED_FACE ( 'NONE', ( #39310, #6544 ), #67409, .F. ) ;
#14922=CARTESIAN_POINT ( 'NONE',  ( 186.5885416670080872, -6.551208109652273848, -3.782341765625003571 ) ) ;
#14975=CARTESIAN_POINT ( 'NONE',  ( 108.3418390382325924, 5.855766388782937426, -5.000000000000004441 ) ) ;
#15016=CARTESIAN_POINT ( 'NONE',  ( 129.5000000000000000, 0.000000000000000000, -6.000000000000000000 ) ) ;
#15098=EDGE_CURVE ( 'NONE', #86875, #69479, #72610, .T. ) ;
#15103=DIRECTION ( 'NONE',  ( 0.000000000000000000, 1.000000000000000000, -1.224646799147353207E-16 ) ) ;
#15221=CARTESIAN_POINT ( 'NONE',  ( 184.6718750003414016, 9.264065473108010111E-16, -7.564683531250000925 ) ) ;
#15226=FACE_OUTER_BOUND ( 'NONE', #39324, .T. ) ;
#15402=CARTESIAN_POINT ( 'NONE',  ( 179.5000000000000000, 0.000000000000000000, 0.000000000000000000 ) ) ;
#15435=DIRECTION ( 'NONE',  ( 0.000000000000000000, 0.000000000000000000, -1.000000000000000000 ) ) ;
#15442=FACE_OUTER_BOUND ( 'NONE', #32424, .T. ) ;
#15457=CARTESIAN_POINT ( 'NONE',  ( 186.9583333333332860, 4.445597072760133273, 7.699999999999975309 ) ) ;
#15458=CARTESIAN_POINT ( 'NONE',  ( 129.5000000000000000, 1.500000000000000000, -2.598076211353316900 ) ) ;
#15467=ORIENTED_EDGE ( 'NONE', *, *, #43250, .F. ) ;
#15477=CARTESIAN_POINT ( 'NONE',  ( 185.3229166673494888, -4.445597072760122614, 7.699999999999998401 ) ) ;
#15492=ORIENTED_EDGE ( 'NONE', *, *, #20761, .T. ) ;
#15520=CARTESIAN_POINT ( 'NONE',  ( 185.8802083336747444, 4.367472073101515306, 7.564683531250000925 ) ) ;
#15546=ORIENTED_EDGE ( 'NONE', *, *, #28290, .F. ) ;
#15591=DIRECTION ( 'NONE',  ( 0.000000000000000000, 0.000000000000000000, 1.000000000000000000 ) ) ;
#15645=LINE ( 'NONE', #66689, #107865 ) ;
#15654=CARTESIAN_POINT ( 'NONE',  ( 129.5000000000000000, -1.375000000000000000, 7.634788798650553154 ) ) ;
#15661=VERTEX_POINT ( 'NONE', #84184 ) ;
#15719=EDGE_CURVE ( 'NONE', #2171, #66080, #68281, .T. ) ;
#15731=ORIENTED_EDGE ( 'NONE', *, *, #85065, .F. ) ;
#15749=AXIS2_PLACEMENT_3D ( 'NONE', #92783, #54141, #53505 ) ;
#15797=CARTESIAN_POINT ( 'NONE',  ( 187.5000000000000000, 0.000000000000000000, 0.000000000000000000 ) ) ;
#15804=VERTEX_POINT ( 'NONE', #9988 ) ;
#15805=PLANE ( 'NONE',  #90997 ) ;
#15832=CARTESIAN_POINT ( 'NONE',  ( 185.0312500006828031, 9.429780353434619030E-16, -7.700000000000000178 ) ) ;
#15864=CARTESIAN_POINT ( 'NONE',  ( 187.5000000000000000, 0.9999999999999985567, 7.634788798650556707 ) ) ;
#15882=CARTESIAN_POINT ( 'NONE',  ( 185.3333333333333144, 6.668395609140177704, -3.849999999999998312 ) ) ;
#15994=CARTESIAN_POINT ( 'NONE',  ( 186.0833333333333144, -6.668395609140180369, 3.849999999999994760 ) ) ;
#16011=CARTESIAN_POINT ( 'NONE',  ( 179.5000000000000000, -1.375000000000000000, 7.634788798650553154 ) ) ;
#16108=CARTESIAN_POINT ( 'NONE',  ( 184.8645833340161175, -6.668395609140180369, 3.849999999999994760 ) ) ;
#16116=AXIS2_PLACEMENT_3D ( 'NONE', #10712, #119391, #79494 ) ;
#16128=CARTESIAN_POINT ( 'NONE',  ( 129.5000000000000000, 0.000000000000000000, 0.000000000000000000 ) ) ;
#16151=CARTESIAN_POINT ( 'NONE',  ( 184.2552083336747444, 6.551208109652275624, -3.782341765624998686 ) ) ;
#16225=CARTESIAN_POINT ( 'NONE',  ( 185.3802083336747444, 4.367472073101515306, 7.564683531250000925 ) ) ;
#16283=VERTEX_POINT ( 'NONE', #92851 ) ;
#16286=DIRECTION ( 'NONE',  ( 0.000000000000000000, 1.000000000000000000, 0.000000000000000000 ) ) ;
#16429=CARTESIAN_POINT ( 'NONE',  ( 127.5000000000000000, -1.500000000000000000, -6.000000000000000000 ) ) ;
#16433=LINE ( 'NONE', #77951, #45213 ) ;
#16515=CARTESIAN_POINT ( 'NONE',  ( 186.8750000000000284, 8.891194145520236347, 5.444286225454521982E-16 ) ) ;
#16541=EDGE_CURVE ( 'NONE', #125237, #51279, #34108, .T. ) ;
#16557=VERTEX_POINT ( 'NONE', #93667 ) ;
#16632=VERTEX_POINT ( 'NONE', #45219 ) ;
#16637=CARTESIAN_POINT ( 'NONE',  ( 109.3185023437525132, 7.233626197500669264, -4.834355238544921995 ) ) ;
#16651=DIRECTION ( 'NONE',  ( 0.000000000000000000, 1.000000000000000000, -1.846105847067148761E-16 ) ) ;
#16750=DIRECTION ( 'NONE',  ( -1.000000000000000000, -0.000000000000000000, -0.000000000000000000 ) ) ;
#16754=CARTESIAN_POINT ( 'NONE',  ( 187.0677083336747444, -4.367472073101514418, -7.564683531250002702 ) ) ;
#16813=CARTESIAN_POINT ( 'NONE',  ( 187.5000000000000000, 1.375000000000002442, -7.576237522675751457 ) ) ;
#16827=CARTESIAN_POINT ( 'NONE',  ( 129.5000000000000000, 0.6250000000000003331, 6.000000000000000000 ) ) ;
#16856=CARTESIAN_POINT ( 'NONE',  ( 185.4218750003414016, 0.000000000000000000, 7.564683531250000925 ) ) ;
#16895=LINE ( 'NONE', #26118, #20120 ) ;
#16923=SHAPE_DEFINITION_REPRESENTATION ( #73316, #5058 ) ;
#16925=CARTESIAN_POINT ( 'NONE',  ( 187.2500000000000000, 9.429780353434619030E-16, -7.700000000000000178 ) ) ;
#16933=LINE ( 'NONE', #118393, #96753 ) ;
#17032=CARTESIAN_POINT ( 'NONE',  ( 185.7812500006828031, 0.000000000000000000, 7.700000000000000178 ) ) ;
#17097=CARTESIAN_POINT ( 'NONE',  ( 129.5000000000000000, -0.6250000000000028866, -7.634788798650553154 ) ) ;
#17140=CARTESIAN_POINT ( 'NONE',  ( 184.2500000000000000, 9.429780353434619030E-16, -7.700000000000000178 ) ) ;
#17278=DIRECTION ( 'NONE',  ( -0.4999999999999471534, -0.000000000000000000, -0.8660254037844692387 ) ) ;
#17345=ORIENTED_EDGE ( 'NONE', *, *, #62717, .F. ) ;
#17398=VECTOR ( 'NONE', #82107, 1000.000000000000000 ) ;
#17402=CARTESIAN_POINT ( 'NONE',  ( 187.2343750003414016, 8.734944146203032389, 5.348610694689227483E-16 ) ) ;
#17475=CARTESIAN_POINT ( 'NONE',  ( 185.2916666666666572, 4.445597072760072876, -7.700000000000080114 ) ) ;
#17509=AXIS2_PLACEMENT_3D ( 'NONE', #3027, #25215, #24591 ) ;
#17525=CARTESIAN_POINT ( 'NONE',  ( 184.0468750003414300, -8.734944146203032389, -1.604583208406767949E-15 ) ) ;
#17547=FACE_OUTER_BOUND ( 'NONE', #72631, .T. ) ;
#17633=ORIENTED_EDGE ( 'NONE', *, *, #96435, .T. ) ;
#17812=CARTESIAN_POINT ( 'NONE',  ( 185.2083333333333144, -4.445597072760115509, -7.700000000000001954 ) ) ;
#17946=CARTESIAN_POINT ( 'NONE',  ( 110.5217483863200414, 7.548960721389698314, -4.329587527523654167 ) ) ;
#17954=ORIENTED_EDGE ( 'NONE', *, *, #24758, .T. ) ;
#17988=ORIENTED_EDGE ( 'NONE', *, *, #82659, .T. ) ;
#18015=CARTESIAN_POINT ( 'NONE',  ( 184.9583333333332860, 4.445597072760175905, 7.699999999999896261 ) ) ;
#18034=CARTESIAN_POINT ( 'NONE',  ( 129.5000000000000000, 1.375000000000000000, 7.576237522675751457 ) ) ;
#18058=CARTESIAN_POINT ( 'NONE',  ( 183.9010416670080588, -4.367472073101519747, 7.564683531249999149 ) ) ;
#18092=VERTEX_POINT ( 'NONE', #128979 ) ;
#18196=DIRECTION ( 'NONE',  ( 0.000000000000000000, 0.000000000000000000, 1.000000000000000000 ) ) ;
#18319=CARTESIAN_POINT ( 'NONE',  ( 127.5000000000000000, -1.500000000000000000, 6.000000000000000000 ) ) ;
#18334=PLANE ( 'NONE',  #46882 ) ;
#18425=VECTOR ( 'NONE', #9878, 1000.000000000000000 ) ;
#18467=CARTESIAN_POINT ( 'NONE',  ( 185.7916666666666572, 4.445597072760120838, -7.699999999999998401 ) ) ;
#18474=CARTESIAN_POINT ( 'NONE',  ( 187.5000000000000000, 0.000000000000000000, 0.000000000000000000 ) ) ;
#18512=CARTESIAN_POINT ( 'NONE',  ( 186.7760416670080588, 6.551208109652274736, 3.782341765625001351 ) ) ;
#18515=CARTESIAN_POINT ( 'NONE',  ( 103.0082443037310611, 8.695253764606311719, -0.3321859063348441832 ) ) ;
#18709=CARTESIAN_POINT ( 'NONE',  ( 185.2343750003414016, 8.734944146203032389, 5.348610694689227483E-16 ) ) ;
#18742=LINE ( 'NONE', #78974, #80357 ) ;
#18769=EDGE_CURVE ( 'NONE', #111172, #26322, #54101, .T. ) ;
#18820=CARTESIAN_POINT ( 'NONE',  ( 186.1302083336747444, -4.367472073101514418, -7.564683531250002702 ) ) ;
#18850=LINE ( 'NONE', #128847, #39335 ) ;
#18900=CARTESIAN_POINT ( 'NONE',  ( 185.9010416670080303, -4.367472073101519747, 7.564683531249999149 ) ) ;
#18908=DIRECTION ( 'NONE',  ( 1.000000000000000000, 0.000000000000000000, 0.000000000000000000 ) ) ;
#18975=DIRECTION ( 'NONE',  ( 1.000000000000000000, 0.000000000000000000, 0.000000000000000000 ) ) ;
#18986=DIRECTION ( 'NONE',  ( -1.000000000000000000, 0.000000000000000000, 0.000000000000000000 ) ) ;
#19068=B_SPLINE_CURVE_WITH_KNOTS ( 'NONE', 3,
 ( #126626, #117404, #116140, #16637, #27758, #67681, #17946, #97795, #48065, #87952, #28424, #108257, #20535, #80750, #38914, #60477, #59179, #69624, #40178, #99099, #49368, #50628, #99745, #90550, #58537, #9422, #113247, #888, #40837, #8750, #88623, #81397, #120022, #10065, #50012, #19894, #120666, #31019, #98423, #70921 ),
 .UNSPECIFIED., .F., .F.,
 ( 4, 2, 2, 2, 2, 2, 2, 2, 2, 2, 2, 2, 2, 2, 2, 2, 2, 2, 2, 4 ),
 ( 0.000000000000000000, 0.0009998201928524694596, 0.001999640385704938919, 0.002999460578557408812, 0.003999280771409877838, 0.004999100964262348165, 0.005998921157114817625, 0.006998741349967286217, 0.007998561542819755676, 0.008498471639245989973, 0.008998381735672226003, 0.009498291832098460299, 0.009998201928524696330, 0.01099802212137718053, 0.01199784231422966647, 0.01299766250708215241, 0.01399748269993463662, 0.01449739279636087959, 0.01499730289278712082, 0.01599712308563960503 ),
 .UNSPECIFIED. ) ;
#19118=ORIENTED_EDGE ( 'NONE', *, *, #60247, .F. ) ;
#19135=CARTESIAN_POINT ( 'NONE',  ( 103.1653408115099211, 8.605869126093731225, -1.317692694826197775 ) ) ;
#19173=UNCERTAINTY_MEASURE_WITH_UNIT (LENGTH_MEASURE( 1.000000000000000082E-05 ), #127086, 'distance_accuracy_value', 'NONE');
#19197=( BOUNDED_CURVE ( )  B_SPLINE_CURVE ( 2, ( #20877, #10404, #90898, #61462, #50336, #49709, #100708 ),
 .UNSPECIFIED., .F., .F. ) 
 B_SPLINE_CURVE_WITH_KNOTS ( ( 3, 2, 2, 3 ),
 ( 0.2857142857142859760, 0.3095238095238098119, 0.3333333333333335924, 0.3571428571428574283 ),
 .UNSPECIFIED. ) 
 CURVE ( )  GEOMETRIC_REPRESENTATION_ITEM ( )  RATIONAL_B_SPLINE_CURVE ( ( 0.9999999999999984457, 0.8660254037844402619, 1.000000000000000000, 0.8660254037844387076, 1.000000000000000000, 0.8660254037844371533, 1.000000000000001554 ) ) 
 REPRESENTATION_ITEM ( '' )  );
#19210=DIRECTION ( 'NONE',  ( -1.000000000000000000, -0.000000000000000000, -0.000000000000000000 ) ) ;
#19256=CARTESIAN_POINT ( 'NONE',  ( 184.3333333333333144, 6.668395609140177704, -3.849999999999998312 ) ) ;
#19343=CARTESIAN_POINT ( 'NONE',  ( 184.2343750003414016, 8.734944146203032389, 5.348610694689227483E-16 ) ) ;
#19361=DIRECTION ( 'NONE',  ( 1.000000000000000000, 0.000000000000000000, 0.000000000000000000 ) ) ;
#19558=CARTESIAN_POINT ( 'NONE',  ( 186.2343750003414016, 8.734944146203032389, 5.348610694689227483E-16 ) ) ;
#19614=CARTESIAN_POINT ( 'NONE',  ( 187.4166666666666856, 6.668395609140176816, 3.850000000000000977 ) ) ;
#19639=DIRECTION ( 'NONE',  ( 0.000000000000000000, -0.000000000000000000, 1.000000000000000000 ) ) ;
#19706=CARTESIAN_POINT ( 'NONE',  ( 185.7916666666666856, 4.445597072760072876, -7.700000000000080114 ) ) ;
#19798=VECTOR ( 'NONE', #31337, 1000.000000000000000 ) ;
#19855=ORIENTED_EDGE ( 'NONE', *, *, #83231, .T. ) ;
#19872=VERTEX_POINT ( 'NONE', #53784 ) ;
#19894=CARTESIAN_POINT ( 'NONE',  ( 109.3219936376940495, 7.239736399353564167, 4.824898011458333968 ) ) ;
#19995=( BOUNDED_CURVE ( )  B_SPLINE_CURVE ( 2, ( #58438, #119265, #118624, #40076, #57127, #49911, #88512 ),
 .UNSPECIFIED., .F., .F. ) 
 B_SPLINE_CURVE_WITH_KNOTS ( ( 3, 2, 2, 3 ),
 ( 0.5000000000000004441, 0.5238095238095242800, 0.5476190476190482270, 0.5714285714285719520 ),
 .UNSPECIFIED. ) 
 CURVE ( )  GEOMETRIC_REPRESENTATION_ITEM ( )  RATIONAL_B_SPLINE_CURVE ( ( 0.9999999999999974465, 0.8660254037844412611, 1.000000000000000000, 0.8660254037844387076, 1.000000000000000000, 0.8660254037844355990, 1.000000000000003109 ) ) 
 REPRESENTATION_ITEM ( '' )  );
#20015=CARTESIAN_POINT ( 'NONE',  ( 185.7760416670080588, 6.551208109652274736, 3.782341765625001351 ) ) ;
#20051=DIRECTION ( 'NONE',  ( -1.000000000000000000, -0.000000000000000000, -0.000000000000000000 ) ) ;
#20120=VECTOR ( 'NONE', #96767, 1000.000000000000000 ) ;
#20165=CARTESIAN_POINT ( 'NONE',  ( 112.9585241711788512, 7.673121854575822631, 0.6644401856000232698 ) ) ;
#20207=CARTESIAN_POINT ( 'NONE',  ( 185.1510416670080872, 4.367472073101518859, -7.564683531249999149 ) ) ;
#20363=EDGE_CURVE ( 'NONE', #4736, #5250, #94681, .T. ) ;
#20378=CARTESIAN_POINT ( 'NONE',  ( 186.4166666666666856, 6.668395609140176816, 3.850000000000000977 ) ) ;
#20459=CARTESIAN_POINT ( 'NONE',  ( 104.6937551430669089, 7.847315309856959686, 3.764367982486338526 ) ) ;
#20521=CARTESIAN_POINT ( 'NONE',  ( 187.5000000000000000, 9.429780353434619030E-16, -7.700000000000000178 ) ) ;
#20535=CARTESIAN_POINT ( 'NONE',  ( 112.4783714810219806, 8.410376606499987417, -2.247359121523905490 ) ) ;
#20548=DIRECTION ( 'NONE',  ( 1.000000000000000000, 0.000000000000000000, 0.000000000000000000 ) ) ;
#20563=CARTESIAN_POINT ( 'NONE',  ( 186.2968750003414584, 8.734944146203032389, 5.348610694689227483E-16 ) ) ;
#20574=( GEOMETRIC_REPRESENTATION_CONTEXT ( 3 ) GLOBAL_UNCERTAINTY_ASSIGNED_CONTEXT ( ( #89864 ) ) GLOBAL_UNIT_ASSIGNED_CONTEXT ( ( #26307, #29522, #69430 ) ) REPRESENTATION_CONTEXT ( 'NONE', 'WORKASPACE' ) );
#20658=CARTESIAN_POINT ( 'NONE',  ( 184.3593750003413732, 0.000000000000000000, 7.564683531250000925 ) ) ;
#20743=CYLINDRICAL_SURFACE ( 'NONE', #81993, 5.000000000000004441 ) ;
#20761=EDGE_CURVE ( 'NONE', #68129, #119603, #59631, .T. ) ;
#20877=CARTESIAN_POINT ( 'NONE',  ( 186.2812500006828031, 0.000000000000000000, 7.700000000000000178 ) ) ;
#20887=EDGE_LOOP ( 'NONE', ( #62568, #9907, #34876, #27049, #46775, #88866, #993, #62239 ) ) ;
#20903=ORIENTED_EDGE ( 'NONE', *, *, #127473, .T. ) ;
#20926=EDGE_CURVE ( 'NONE', #110378, #15661, #123042, .T. ) ;
#21071=EDGE_CURVE ( 'NONE', #49367, #114625, #106605, .T. ) ;
#21079=EDGE_LOOP ( 'NONE', ( #105650, #86901, #51284, #9718, #111532, #35065, #25327 ) ) ;
#21086=CARTESIAN_POINT ( 'NONE',  ( 186.1510416670080588, 4.367472073101518859, -7.564683531249999149 ) ) ;
#21108=LINE ( 'NONE', #61034, #58439 ) ;
#21151=CIRCLE ( 'NONE', #96355, 7.700000000000000178 ) ;
#21291=DIRECTION ( 'NONE',  ( -1.000000000000000000, -0.000000000000000000, -0.000000000000000000 ) ) ;
#21405=VECTOR ( 'NONE', #30828, 1000.000000000000000 ) ;
#21412=DIRECTION ( 'NONE',  ( -1.000000000000000000, -0.000000000000000000, -0.000000000000000000 ) ) ;
#21460=ORIENTED_EDGE ( 'NONE', *, *, #35659, .F. ) ;
#21491=CARTESIAN_POINT ( 'NONE',  ( 187.4218750003414016, 0.000000000000000000, 7.564683531250000925 ) ) ;
#21529=ORIENTED_EDGE ( 'NONE', *, *, #37666, .F. ) ;
#21537=ORIENTED_EDGE ( 'NONE', *, *, #77501, .F. ) ;
#21586=VECTOR ( 'NONE', #67734, 1000.000000000000000 ) ;
#21592=EDGE_CURVE ( 'NONE', #94263, #102067, #65884, .T. ) ;
#21604=EDGE_CURVE ( 'NONE', #49367, #21810, #96001, .T. ) ;
#21642=DIRECTION ( 'NONE',  ( 1.000000000000000000, 0.000000000000000000, 0.000000000000000000 ) ) ;
#21729=AXIS2_PLACEMENT_3D ( 'NONE', #25406, #66629, #29304 ) ;
#21738=DIRECTION ( 'NONE',  ( 0.000000000000000000, 1.000000000000000000, -0.000000000000000000 ) ) ;
#21746=CARTESIAN_POINT ( 'NONE',  ( 186.2343750003414016, 8.734944146203032389, 5.348610694689227483E-16 ) ) ;
#21802=VECTOR ( 'NONE', #119781, 1000.000000000000000 ) ;
#21810=VERTEX_POINT ( 'NONE', #107090 ) ;
#21838=EDGE_CURVE ( 'NONE', #111172, #77053, #101808, .T. ) ;
#21849=DIRECTION ( 'NONE',  ( 0.000000000000000000, 0.000000000000000000, -1.000000000000000000 ) ) ;
#21864=CARTESIAN_POINT ( 'NONE',  ( 186.5885416670080872, -6.551208109652273848, -3.782341765625003571 ) ) ;
#22007=CARTESIAN_POINT ( 'NONE',  ( 187.5000000000000000, 0.000000000000000000, 0.000000000000000000 ) ) ;
#22116=CARTESIAN_POINT ( 'NONE',  ( 185.9062500006828316, -8.891194145520236347, -1.633285867636356693E-15 ) ) ;
#22162=CARTESIAN_POINT ( 'NONE',  ( 184.2760416670080588, 6.551208109652274736, 3.782341765625001351 ) ) ;
#22270=ORIENTED_EDGE ( 'NONE', *, *, #88137, .F. ) ;
#22288=CARTESIAN_POINT ( 'NONE',  ( 103.0088460997482400, 7.694247472631703388, 0.3420374265531280211 ) ) ;
#22402=CARTESIAN_POINT ( 'NONE',  ( 184.5677083336747444, -4.367472073101514418, -7.564683531250002702 ) ) ;
#22469=ORIENTED_EDGE ( 'NONE', *, *, #51756, .F. ) ;
#22528=EDGE_CURVE ( 'NONE', #114300, #1392, #49675, .T. ) ;
#22545=ORIENTED_EDGE ( 'NONE', *, *, #38255, .F. ) ;
#22548=CARTESIAN_POINT ( 'NONE',  ( 183.9479166673494603, -6.668395609140176816, -3.850000000000003642 ) ) ;
#22610=ORIENTED_EDGE ( 'NONE', *, *, #31488, .T. ) ;
#22685=DIRECTION ( 'NONE',  ( 0.000000000000000000, 0.000000000000000000, 1.000000000000000000 ) ) ;
#22691=LINE ( 'NONE', #102518, #102240 ) ;
#22804=CARTESIAN_POINT ( 'NONE',  ( 187.3802083336747444, 4.367472073101515306, 7.564683531250000925 ) ) ;
#22856=CARTESIAN_POINT ( 'NONE',  ( 179.5000000000000000, 1.375000000000002442, -6.000000000000000888 ) ) ;
#22870=CYLINDRICAL_SURFACE ( 'NONE', #88086, 7.700000000000000178 ) ;
#22873=EDGE_LOOP ( 'NONE', ( #56439, #75412, #6916, #106820 ) ) ;
#22884=CARTESIAN_POINT ( 'NONE',  ( 179.5000000000000000, 0.9999999999999985567, 7.634788798650556707 ) ) ;
#22891=VECTOR ( 'NONE', #49391, 1000.000000000000000 ) ;
#22930=CARTESIAN_POINT ( 'NONE',  ( 184.7812500006828031, 0.000000000000000000, 7.700000000000000178 ) ) ;
#22968=CARTESIAN_POINT ( 'NONE',  ( 129.5000000000000000, -1.500000000000000000, 2.598076211353316900 ) ) ;
#23021=ADVANCED_FACE ( 'NONE', ( #128062, #28573 ), #38412, .T. ) ;
#23025=EDGE_CURVE ( 'NONE', #113580, #111172, #18742, .T. ) ;
#23094=SURFACE_STYLE_FILL_AREA ( #64931 ) ;
#23096=CARTESIAN_POINT ( 'NONE',  ( 186.2812500006828031, 0.000000000000000000, 7.700000000000000178 ) ) ;
#23112=EDGE_LOOP ( 'NONE', ( #42039, #58868, #36116, #76853 ) ) ;
#23132=CARTESIAN_POINT ( 'NONE',  ( 187.0833333333333144, -6.668395609140180369, 3.849999999999994760 ) ) ;
#23165=VERTEX_POINT ( 'NONE', #63185 ) ;
#23174=DIRECTION ( 'NONE',  ( 0.000000000000000000, 0.000000000000000000, 1.000000000000000000 ) ) ;
#23181=ORIENTED_EDGE ( 'NONE', *, *, #10603, .T. ) ;
#23301=CARTESIAN_POINT ( 'NONE',  ( 187.3333333333333144, 6.668395609140177704, -3.849999999999998312 ) ) ;
#23360=CARTESIAN_POINT ( 'NONE',  ( 187.1979166673494603, 6.668395609140176816, 3.850000000000000977 ) ) ;
#23412=CARTESIAN_POINT ( 'NONE',  ( 186.5885416670080872, -6.551208109652273848, -3.782341765625003571 ) ) ;
#23508=CARTESIAN_POINT ( 'NONE',  ( 186.6145833340161175, 6.668395609140177704, -3.849999999999998312 ) ) ;
#23546=CARTESIAN_POINT ( 'NONE',  ( 104.6974693483957282, 6.720082114647700777, -3.767527145165660674 ) ) ;
#23575=CARTESIAN_POINT ( 'NONE',  ( 187.5000000000000000, 0.000000000000000000, 0.000000000000000000 ) ) ;
#23579=CARTESIAN_POINT ( 'NONE',  ( 185.9062500006827747, -8.891194145520236347, -1.633285867636356299E-15 ) ) ;
#23583=LINE ( 'NONE', #25504, #10152 ) ;
#23671=CARTESIAN_POINT ( 'NONE',  ( 185.2343750003414016, 8.734944146203032389, 5.348610694689227483E-16 ) ) ;
#23725=CARTESIAN_POINT ( 'NONE',  ( 129.5000000000000000, 1.375000000000000000, 7.634788798650556707 ) ) ;
#23787=CARTESIAN_POINT ( 'NONE',  ( 184.0468750003414300, -8.734944146203032389, -1.604583208406768146E-15 ) ) ;
#23816=CARTESIAN_POINT ( 'NONE',  ( 186.5833333333333144, -6.668395609140180369, 3.849999999999994760 ) ) ;
#23898=CARTESIAN_POINT ( 'NONE',  ( 184.5833333333333144, -6.668395609140180369, 3.849999999999994760 ) ) ;
#23910=DIRECTION ( 'NONE',  ( -1.000000000000000000, -0.000000000000000000, -0.000000000000000000 ) ) ;
#23962=ADVANCED_FACE ( 'NONE', ( #26981, #109391 ), #99589, .T. ) ;
#23975=EDGE_CURVE ( 'NONE', #50117, #38386, #42563, .T. ) ;
#24075=CARTESIAN_POINT ( 'NONE',  ( 184.1510416670080588, 4.367472073101518859, -7.564683531249999149 ) ) ;
#24113=CARTESIAN_POINT ( 'NONE',  ( 184.7500000000000000, 9.429780353434619030E-16, -7.700000000000000178 ) ) ;
#24143=CARTESIAN_POINT ( 'NONE',  ( 187.3385416670080872, 6.551208109652274736, 3.782341765625001351 ) ) ;
#24146=DIRECTION ( 'NONE',  ( 0.000000000000000000, -1.846105847067148515E-16, -1.000000000000000000 ) ) ;
#24203=CARTESIAN_POINT ( 'NONE',  ( 106.6633797337217970, 5.997582082682869853, -4.829774833287197922 ) ) ;
#24373=ORIENTED_EDGE ( 'NONE', *, *, #28290, .T. ) ;
#24396=ORIENTED_EDGE ( 'NONE', *, *, #21592, .T. ) ;
#24423=CARTESIAN_POINT ( 'NONE',  ( 184.8385416670080872, 6.551208109652274736, 3.782341765625001351 ) ) ;
#24430=EDGE_CURVE ( 'NONE', #57186, #79091, #109029, .T. ) ;
#24512=ORIENTED_EDGE ( 'NONE', *, *, #83551, .F. ) ;
#24531=CARTESIAN_POINT ( 'NONE',  ( 184.7083333333333428, -4.445597072760175017, -7.699999999999898037 ) ) ;
#24559=EDGE_LOOP ( 'NONE', ( #36919, #34579, #3426, #104820 ) ) ;
#24591=DIRECTION ( 'NONE',  ( 0.000000000000000000, 0.000000000000000000, 1.000000000000000000 ) ) ;
#24597=EDGE_CURVE ( 'NONE', #63648, #90185, #2711, .T. ) ;
#24653=LINE ( 'NONE', #64564, #70392 ) ;
#24680=ORIENTED_EDGE ( 'NONE', *, *, #77501, .T. ) ;
#24714=VECTOR ( 'NONE', #14854, 1000.000000000000000 ) ;
#24719=CARTESIAN_POINT ( 'NONE',  ( 185.3802083336747160, 4.367472073101515306, 7.564683531250000925 ) ) ;
#24756=DIRECTION ( 'NONE',  ( 0.000000000000000000, 0.000000000000000000, 1.000000000000000000 ) ) ;
#24758=EDGE_CURVE ( 'NONE', #117106, #80059, #90296, .T. ) ;
#24787=CARTESIAN_POINT ( 'NONE',  ( 186.7135416670080872, 4.367472073101518859, -7.564683531249999149 ) ) ;
#24794=ORIENTED_EDGE ( 'NONE', *, *, #22528, .F. ) ;
#24801=CIRCLE ( 'NONE', #68703, 7.700000000000000178 ) ;
#24871=AXIS2_PLACEMENT_3D ( 'NONE', #53361, #93278, #72993 ) ;
#24972=VECTOR ( 'NONE', #48646, 1000.000000000000000 ) ;
#25043=EDGE_LOOP ( 'NONE', ( #19855, #102100, #119465, #34152 ) ) ;
#25066=CARTESIAN_POINT ( 'NONE',  ( 184.1718750003414016, 9.264065473108010111E-16, -7.564683531250000925 ) ) ;
#25164=ORIENTED_EDGE ( 'NONE', *, *, #10553, .F. ) ;
#25215=DIRECTION ( 'NONE',  ( -1.000000000000000000, -0.000000000000000000, -0.000000000000000000 ) ) ;
#25290=CARTESIAN_POINT ( 'NONE',  ( 183.8645833340161175, -6.668395609140180369, 3.849999999999994760 ) ) ;
#25299=CARTESIAN_POINT ( 'NONE',  ( 129.5000000000000000, 1.375000000000000000, 7.634788798650556707 ) ) ;
#25318=EDGE_CURVE ( 'NONE', #119603, #9738, #109474, .T. ) ;
#25327=ORIENTED_EDGE ( 'NONE', *, *, #115199, .T. ) ;
#25329=CARTESIAN_POINT ( 'NONE',  ( 185.5416666666666856, -4.445597072760063107, 7.700000000000102318 ) ) ;
#25332=CARTESIAN_POINT ( 'NONE',  ( 129.5000000000000000, 0.000000000000000000, 0.000000000000000000 ) ) ;
#25406=CARTESIAN_POINT ( 'NONE',  ( 187.5000000000000000, 0.000000000000000000, 0.000000000000000000 ) ) ;
#25421=VECTOR ( 'NONE', #21412, 1000.000000000000000 ) ;
#25452=CARTESIAN_POINT ( 'NONE',  ( 108.0000000000000142, 5.855766388782936538, -5.000000000000004441 ) ) ;
#25460=PRODUCT_DEFINITION_FORMATION_WITH_SPECIFIED_SOURCE ( 'ANY', '', #57498, .NOT_KNOWN. ) ;
#25466=VECTOR ( 'NONE', #2798, 1000.000000000000000 ) ;
#25480=LINE ( 'NONE', #15654, #107545 ) ;
#25481=VECTOR ( 'NONE', #95004, 1000.000000000000000 ) ;
#25504=CARTESIAN_POINT ( 'NONE',  ( 187.5000000000000000, 0.000000000000000000, 7.700000000000000178 ) ) ;
#25615=CYLINDRICAL_SURFACE ( 'NONE', #7959, 7.700000000000000178 ) ;
#25647=EDGE_CURVE ( 'NONE', #86071, #33663, #28188, .T. ) ;
#25678=ORIENTED_EDGE ( 'NONE', *, *, #55526, .F. ) ;
#25707=CARTESIAN_POINT ( 'NONE',  ( 187.4166666666666856, 6.668395609140176816, 3.850000000000000977 ) ) ;
#25711=DIRECTION ( 'NONE',  ( 0.000000000000000000, 0.000000000000000000, 1.000000000000000000 ) ) ;
#25715=DIRECTION ( 'NONE',  ( 1.000000000000000000, 0.000000000000000000, 0.000000000000000000 ) ) ;
#25965=CARTESIAN_POINT ( 'NONE',  ( 187.2760416670080588, 6.551208109652274736, 3.782341765625001351 ) ) ;
#26011=CARTESIAN_POINT ( 'NONE',  ( 185.0885416670080872, -6.551208109652273848, -3.782341765625003571 ) ) ;
#26070=ADVANCED_FACE ( 'NONE', ( #17547 ), #120759, .F. ) ;
#26079=EDGE_CURVE ( 'NONE', #117106, #85617, #67944, .T. ) ;
#26080=CARTESIAN_POINT ( 'NONE',  ( 185.6718750003414016, 9.264065473108010111E-16, -7.564683531250000925 ) ) ;
#26083=FACE_OUTER_BOUND ( 'NONE', #23112, .T. ) ;
#26118=CARTESIAN_POINT ( 'NONE',  ( 187.3906250003414016, 0.000000000000000000, 7.700000000000000178 ) ) ;
#26307=( LENGTH_UNIT ( ) NAMED_UNIT ( * ) SI_UNIT ( .MILLI., .METRE. ) );
#26322=VERTEX_POINT ( 'NONE', #102415 ) ;
#26368=CARTESIAN_POINT ( 'NONE',  ( 185.0000000000000000, 0.000000000000000000, 7.700000000000000178 ) ) ;
#26602=LINE ( 'NONE', #66511, #63724 ) ;
#26604=CARTESIAN_POINT ( 'NONE',  ( 184.6562500006828031, 8.891194145520236347, 5.444286225454521982E-16 ) ) ;
#26650=CARTESIAN_POINT ( 'NONE',  ( 185.6718750003414016, 9.264065473108010111E-16, -7.564683531250000925 ) ) ;
#26701=EDGE_LOOP ( 'NONE', ( #70362, #46423, #80679, #24396 ) ) ;
#26719=CARTESIAN_POINT ( 'NONE',  ( 185.7968750003414300, 8.734944146203032389, 5.348610694689227483E-16 ) ) ;
#26786=CARTESIAN_POINT ( 'NONE',  ( 187.1666666666666856, -6.668395609140176816, -3.850000000000003642 ) ) ;
#26981=FACE_BOUND ( 'NONE', #98836, .T. ) ;
#27009=CARTESIAN_POINT ( 'NONE',  ( 184.4583333333333428, 4.445597072760117285, 7.699999999999999289 ) ) ;
#27049=ORIENTED_EDGE ( 'NONE', *, *, #63430, .T. ) ;
#27086=CIRCLE ( 'NONE', #35502, 7.700000000000000178 ) ;
#27236=CARTESIAN_POINT ( 'NONE',  ( 184.9895833340161175, -4.445597072760115509, -7.700000000000001954 ) ) ;
#27279=CARTESIAN_POINT ( 'NONE',  ( 185.9218750003414016, 0.000000000000000000, 7.564683531250000925 ) ) ;
#27336=CARTESIAN_POINT ( 'NONE',  ( 186.0885416670080872, -6.551208109652273848, -3.782341765625003571 ) ) ;
#27369=ORIENTED_EDGE ( 'NONE', *, *, #128795, .T. ) ;
#27471=CARTESIAN_POINT ( 'NONE',  ( 187.5000000000000000, 0.000000000000000000, 0.000000000000000000 ) ) ;
#27593=ORIENTED_EDGE ( 'NONE', *, *, #34794, .F. ) ;
#27599=CIRCLE ( 'NONE', #98605, 7.700000000000000178 ) ;
#27623=CARTESIAN_POINT ( 'NONE',  ( 185.8750000000000000, 8.891194145520236347, 5.444286225454521982E-16 ) ) ;
#27736=ORIENTED_EDGE ( 'NONE', *, *, #45844, .F. ) ;
#27758=CARTESIAN_POINT ( 'NONE',  ( 109.6384078294126283, 7.300040591920232913, -4.735138557421405991 ) ) ;
#27777=CARTESIAN_POINT ( 'NONE',  ( 184.0729166673494603, 4.445597072760049784, -7.700000000000123634 ) ) ;
#27809=LINE ( 'NONE', #48761, #21586 ) ;
#27968=VERTEX_POINT ( 'NONE', #72351 ) ;
#28006=CARTESIAN_POINT ( 'NONE',  ( 184.7135416670080588, 4.367472073101518859, -7.564683531249999149 ) ) ;
#28022=EDGE_CURVE ( 'NONE', #12583, #38386, #80875, .T. ) ;
#28092=CARTESIAN_POINT ( 'NONE',  ( 187.2760416670080588, 6.551208109652274736, 3.782341765625001351 ) ) ;
#28167=FACE_OUTER_BOUND ( 'NONE', #29931, .T. ) ;
#28188=LINE ( 'NONE', #100155, #21802 ) ;
#28202=ORIENTED_EDGE ( 'NONE', *, *, #125313, .F. ) ;
#28290=EDGE_CURVE ( 'NONE', #113580, #99802, #88420, .T. ) ;
#28295=CARTESIAN_POINT ( 'NONE',  ( 185.0833333333333144, -6.668395609140180369, 3.849999999999994760 ) ) ;
#28347=CARTESIAN_POINT ( 'NONE',  ( 186.9010416670080588, -4.367472073101520635, 7.564683531249999149 ) ) ;
#28424=CARTESIAN_POINT ( 'NONE',  ( 111.9633609056390071, 8.147017582221319998, -3.065257838783662425 ) ) ;
#28508=VECTOR ( 'NONE', #74044, 1000.000000000000000 ) ;
#28541=CARTESIAN_POINT ( 'NONE',  ( 185.5260416670080588, -6.551208109652273848, -3.782341765625003571 ) ) ;
#28573=FACE_BOUND ( 'NONE', #61024, .T. ) ;
#28661=CARTESIAN_POINT ( 'NONE',  ( 184.9635416670080588, -4.367472073101520635, 7.564683531249999149 ) ) ;
#28681=ORIENTED_EDGE ( 'NONE', *, *, #62605, .F. ) ;
#28706=CARTESIAN_POINT ( 'NONE',  ( 112.4709740538754943, 7.366778627195011531, -2.262163914407335330 ) ) ;
#28747=CARTESIAN_POINT ( 'NONE',  ( 186.4010416670080588, -4.367472073101519747, 7.564683531249999149 ) ) ;
#28848=CARTESIAN_POINT ( 'NONE',  ( 184.5729166673494888, 4.445597072760062218, -7.700000000000102318 ) ) ;
#28878=CARTESIAN_POINT ( 'NONE',  ( 187.5000000000000000, 9.429780353434619030E-16, -7.700000000000000178 ) ) ;
#28950=CARTESIAN_POINT ( 'NONE',  ( 186.6666666666666856, -6.668395609140176816, -3.850000000000003642 ) ) ;
#28952=CARTESIAN_POINT ( 'NONE',  ( 187.4218750003414016, 0.000000000000000000, 7.564683531250000925 ) ) ;
#28984=STYLED_ITEM ( 'NONE', ( #57028 ), #78940 ) ;
#28994=CARTESIAN_POINT ( 'NONE',  ( 186.9427083336747160, -6.551208109652278289, 3.782341765624995134 ) ) ;
#28996=CARTESIAN_POINT ( 'NONE',  ( 104.2436697997757165, 8.047302484776873044, -3.315374049100932474 ) ) ;
#29111=CARTESIAN_POINT ( 'NONE',  ( 179.5000000000000000, -1.000000000000025535, -7.634788798650553154 ) ) ;
#29124=VERTEX_POINT ( 'NONE', #53217 ) ;
#29155=DIRECTION ( 'NONE',  ( 0.000000000000000000, -1.000000000000000000, 0.000000000000000000 ) ) ;
#29201=VECTOR ( 'NONE', #4965, 1000.000000000000000 ) ;
#29202=CARTESIAN_POINT ( 'NONE',  ( 184.4010416670080872, -4.367472073101519747, 7.564683531249999149 ) ) ;
#29304=DIRECTION ( 'NONE',  ( 0.000000000000000000, 0.000000000000000000, 1.000000000000000000 ) ) ;
#29330=EDGE_LOOP ( 'NONE', ( #25678, #75069, #54062, #11713 ) ) ;
#29362=CARTESIAN_POINT ( 'NONE',  ( 129.5000000000000000, 0.000000000000000000, 0.000000000000000000 ) ) ;
#29394=CARTESIAN_POINT ( 'NONE',  ( 185.2760416670080588, 6.551208109652274736, 3.782341765625001351 ) ) ;
#29424=ORIENTED_EDGE ( 'NONE', *, *, #99768, .F. ) ;
#29440=CARTESIAN_POINT ( 'NONE',  ( 187.3750000000000000, 8.891194145520236347, 5.444286225454521982E-16 ) ) ;
#29491=ORIENTED_EDGE ( 'NONE', *, *, #23975, .F. ) ;
#29514=CARTESIAN_POINT ( 'NONE',  ( 106.3595699872024198, 6.079292664285325998, 4.726105526114997346 ) ) ;
#29522=( NAMED_UNIT ( * ) PLANE_ANGLE_UNIT ( ) SI_UNIT ( $, .RADIAN. ) );
#29619=CARTESIAN_POINT ( 'NONE',  ( 186.9843750003414016, -8.734944146203032389, -1.604583208406767949E-15 ) ) ;
#29742=DIRECTION ( 'NONE',  ( -0.000000000000000000, 1.000000000000000000, 1.846105847067148022E-16 ) ) ;
#29769=CARTESIAN_POINT ( 'NONE',  ( 183.8645833340161175, -6.668395609140180369, 3.849999999999994760 ) ) ;
#29829=CARTESIAN_POINT ( 'NONE',  ( 185.1927083336747160, 6.551208109652275624, -3.782341765624998686 ) ) ;
#29931=EDGE_LOOP ( 'NONE', ( #80755, #99152, #117465, #57459 ) ) ;
#29935=ORIENTED_EDGE ( 'NONE', *, *, #223, .T. ) ;
#29997=CARTESIAN_POINT ( 'NONE',  ( 111.0564249898064588, 6.601081615736754671, -3.969972484914319200 ) ) ;
#30012=DIRECTION ( 'NONE',  ( 0.000000000000000000, -1.846105847067148022E-16, 1.000000000000000000 ) ) ;
#30020=ORIENTED_EDGE ( 'NONE', *, *, #56646, .T. ) ;
#30038=CARTESIAN_POINT ( 'NONE',  ( 185.4010416670080588, -4.367472073101519747, 7.564683531249999149 ) ) ;
#30170=LINE ( 'NONE', #28878, #32592 ) ;
#30182=CARTESIAN_POINT ( 'NONE',  ( 186.0000000000000000, 0.000000000000000000, 7.700000000000000178 ) ) ;
#30188=ORIENTED_EDGE ( 'NONE', *, *, #11308, .T. ) ;
#30189=ORIENTED_EDGE ( 'NONE', *, *, #26079, .F. ) ;
#30292=CARTESIAN_POINT ( 'NONE',  ( 186.5677083336747160, -4.367472073101514418, -7.564683531250002702 ) ) ;
#30296=CARTESIAN_POINT ( 'NONE',  ( 105.7603592657142144, 7.458072953931099036, -4.482094334535867475 ) ) ;
#30391=VECTOR ( 'NONE', #108094, 1000.000000000000000 ) ;
#30405=CARTESIAN_POINT ( 'NONE',  ( 186.3802083336747444, 4.367472073101515306, 7.564683531250000925 ) ) ;
#30495=CARTESIAN_POINT ( 'NONE',  ( 184.3177083336747160, 4.367472073101515306, 7.564683531250000925 ) ) ;
#30541=DIRECTION ( 'NONE',  ( -1.000000000000000000, -0.000000000000000000, -0.000000000000000000 ) ) ;
#30665=CARTESIAN_POINT ( 'NONE',  ( 108.0000000000000142, 5.855766388782936538, -5.000000000000004441 ) ) ;
#30688=CARTESIAN_POINT ( 'NONE',  ( 185.4843750003414300, -8.734944146203032389, -1.604583208406768146E-15 ) ) ;
#30820=CARTESIAN_POINT ( 'NONE',  ( 103.7759110461913821, 7.219941590808979015, 2.680022258956899162 ) ) ;
#30828=DIRECTION ( 'NONE',  ( 0.000000000000000000, 1.846105847067148022E-16, -1.000000000000000000 ) ) ;
#30856=CARTESIAN_POINT ( 'NONE',  ( 186.2916666666666288, 4.445597072760091528, -7.700000000000049916 ) ) ;
#30931=CARTESIAN_POINT ( 'NONE',  ( 185.3177083336747160, 4.367472073101515306, 7.564683531250000925 ) ) ;
#30935=CARTESIAN_POINT ( 'NONE',  ( 106.6782762233207507, 7.234168045436613070, -4.833551603070167069 ) ) ;
#31002=VECTOR ( 'NONE', #79351, 1000.000000000000000 ) ;
#31019=CARTESIAN_POINT ( 'NONE',  ( 108.6701129985725487, 7.143859034846247624, 4.966056649218576702 ) ) ;
#31049=CARTESIAN_POINT ( 'NONE',  ( 186.1718750003414016, 9.264065473108010111E-16, -7.564683531250000925 ) ) ;
#31084=( BOUNDED_CURVE ( )  B_SPLINE_CURVE ( 2, ( #68944, #128544, #39518, #78789, #88587, #100984, #9389 ),
 .UNSPECIFIED., .F., .F. ) 
 B_SPLINE_CURVE_WITH_KNOTS ( ( 3, 2, 2, 3 ),
 ( 0.6428571428571433488, 0.6666666666666670737, 0.6904761904761910207, 0.7142857142857148567 ),
 .UNSPECIFIED. ) 
 CURVE ( )  GEOMETRIC_REPRESENTATION_ITEM ( )  RATIONAL_B_SPLINE_CURVE ( ( 0.9999999999999974465, 0.8660254037844412611, 1.000000000000000000, 0.8660254037844387076, 1.000000000000000000, 0.8660254037844355990, 1.000000000000003109 ) ) 
 REPRESENTATION_ITEM ( '' )  );
#31133=VERTEX_POINT ( 'NONE', #51637 ) ;
#31223=CARTESIAN_POINT ( 'NONE',  ( 186.4062500006828031, -8.891194145520236347, -1.633285867636356299E-15 ) ) ;
#31243=DIRECTION ( 'NONE',  ( 0.000000000000000000, 0.000000000000000000, 1.000000000000000000 ) ) ;
#31260=EDGE_CURVE ( 'NONE', #94355, #79874, #59545, .T. ) ;
#31330=APPLICATION_CONTEXT ( 'automotive_design' ) ;
#31331=CARTESIAN_POINT ( 'NONE',  ( 186.5468750003414300, -8.734944146203032389, -1.604583208406768146E-15 ) ) ;
#31337=DIRECTION ( 'NONE',  ( 0.000000000000000000, 0.000000000000000000, -1.000000000000000000 ) ) ;
#31488=EDGE_CURVE ( 'NONE', #127679, #16283, #118610, .T. ) ;
#31563=CARTESIAN_POINT ( 'NONE',  ( 184.2760416670080588, 6.551208109652274736, 3.782341765625001351 ) ) ;
#31596=CARTESIAN_POINT ( 'NONE',  ( 88.00000000000001421, 1.065442715258197248E-15, -8.699999999999999289 ) ) ;
#31625=CARTESIAN_POINT ( 'NONE',  ( 185.2812500006828031, 0.000000000000000000, 7.700000000000000178 ) ) ;
#31669=CARTESIAN_POINT ( 'NONE',  ( 187.1718750003414016, 9.264065473108010111E-16, -7.564683531250000925 ) ) ;
#31692=ORIENTED_EDGE ( 'NONE', *, *, #8159, .T. ) ;
#31783=LINE ( 'NONE', #50146, #3844 ) ;
#31790=ORIENTED_EDGE ( 'NONE', *, *, #912, .T. ) ;
#31852=CARTESIAN_POINT ( 'NONE',  ( 129.5000000000000000, 1.500000000000000000, 0.000000000000000000 ) ) ;
#31917=CARTESIAN_POINT ( 'NONE',  ( 186.3229166673494603, -4.445597072760122614, 7.699999999999998401 ) ) ;
#31926=CIRCLE ( 'NONE', #40234, 7.700000000000000178 ) ;
#31972=CARTESIAN_POINT ( 'NONE',  ( 187.2968750003414300, 8.734944146203032389, 5.348610694689227483E-16 ) ) ;
#32030=ADVANCED_FACE ( 'NONE', ( #41522 ), #81431, .T. ) ;
#32090=CARTESIAN_POINT ( 'NONE',  ( 129.5000000000000000, 0.6250000000000028866, -7.634788798650556707 ) ) ;
#32124=CARTESIAN_POINT ( 'NONE',  ( 187.5000000000000000, 0.9999999999999985567, -7.634788798650556707 ) ) ;
#32136=CARTESIAN_POINT ( 'NONE',  ( 129.5000000000000000, -1.500000000000000000, 6.000000000000000000 ) ) ;
#32185=CARTESIAN_POINT ( 'NONE',  ( 108.0000000000000142, 8.700999999999998735, 5.000000000000004441 ) ) ;
#32212=VECTOR ( 'NONE', #128144, 1000.000000000000000 ) ;
#32225=CARTESIAN_POINT ( 'NONE',  ( 185.1927083336747160, 6.551208109652275624, -3.782341765624998686 ) ) ;
#32252=CARTESIAN_POINT ( 'NONE',  ( 184.3229166673494603, -4.445597072760039126, 7.700000000000142286 ) ) ;
#32262=VECTOR ( 'NONE', #124050, 1000.000000000000000 ) ;
#32341=CARTESIAN_POINT ( 'NONE',  ( 186.3385416670080872, 6.551208109652274736, 3.782341765625001351 ) ) ;
#32424=EDGE_LOOP ( 'NONE', ( #46204, #107506, #15546, #13469 ) ) ;
#32473=CARTESIAN_POINT ( 'NONE',  ( 179.5000000000000000, 0.6250000000000000000, -6.000000000000000000 ) ) ;
#32575=ORIENTED_EDGE ( 'NONE', *, *, #106734, .T. ) ;
#32577=AXIS2_PLACEMENT_3D ( 'NONE', #33653, #103025, #23174 ) ;
#32592=VECTOR ( 'NONE', #1327, 1000.000000000000000 ) ;
#32637=CARTESIAN_POINT ( 'NONE',  ( 183.9843750003414016, -8.734944146203032389, -1.604583208406768146E-15 ) ) ;
#32655=ORIENTED_EDGE ( 'NONE', *, *, #7166, .F. ) ;
#32664=CARTESIAN_POINT ( 'NONE',  ( 187.5000000000000000, 0.000000000000000000, 0.000000000000000000 ) ) ;
#32680=CARTESIAN_POINT ( 'NONE',  ( 87.50000000000001421, 0.000000000000000000, 0.000000000000000000 ) ) ;
#32725=CIRCLE ( 'NONE', #114186, 7.700000000000000178 ) ;
#32770=CARTESIAN_POINT ( 'NONE',  ( 184.9479166673494603, -6.668395609140176816, -3.850000000000003642 ) ) ;
#32796=CARTESIAN_POINT ( 'NONE',  ( 187.2500000000000000, 9.429780353434619030E-16, -7.700000000000000178 ) ) ;
#32868=CARTESIAN_POINT ( 'NONE',  ( 129.5000000000000000, 0.000000000000000000, 0.000000000000000000 ) ) ;
#32870=CARTESIAN_POINT ( 'NONE',  ( 183.9427083336747160, -6.551208109652278289, 3.782341765624995134 ) ) ;
#32940=( NAMED_UNIT ( * ) SI_UNIT ( $, .STERADIAN. ) SOLID_ANGLE_UNIT ( ) );
#32975=CARTESIAN_POINT ( 'NONE',  ( 187.1250000000000284, -8.891194145520236347, -1.633285867636356693E-15 ) ) ;
#33021=DIRECTION ( 'NONE',  ( 0.000000000000000000, -1.846105847067148515E-16, -1.000000000000000000 ) ) ;
#33034=VERTEX_POINT ( 'NONE', #99947 ) ;
#33154=DIRECTION ( 'NONE',  ( 0.000000000000000000, 0.000000000000000000, -1.000000000000000000 ) ) ;
#33155=CARTESIAN_POINT ( 'NONE',  ( 186.2812500006828031, 0.000000000000000000, 7.700000000000000178 ) ) ;
#33221=CARTESIAN_POINT ( 'NONE',  ( 185.5729166673494319, 4.445597072760120838, -7.699999999999998401 ) ) ;
#33268=CARTESIAN_POINT ( 'NONE',  ( 187.0885416670080872, -6.551208109652273848, -3.782341765625003571 ) ) ;
#33284=ORIENTED_EDGE ( 'NONE', *, *, #91538, .F. ) ;
#33314=CARTESIAN_POINT ( 'NONE',  ( 179.5000000000000000, 0.6250000000000025535, -6.000000000000000888 ) ) ;
#33335=ADVANCED_FACE ( 'NONE', ( #66759 ), #44559, .F. ) ;
#33375=ORIENTED_EDGE ( 'NONE', *, *, #76870, .F. ) ;
#33394=CARTESIAN_POINT ( 'NONE',  ( 103.0671989394255945, 7.656491474633341454, -0.8341323537259196508 ) ) ;
#33449=CARTESIAN_POINT ( 'NONE',  ( 187.1562500006828316, 8.891194145520236347, 5.444286225454521982E-16 ) ) ;
#33508=CARTESIAN_POINT ( 'NONE',  ( 185.9427083336747160, -6.551208109652278289, 3.782341765624995134 ) ) ;
#33527=LINE ( 'NONE', #53790, #104482 ) ;
#33535=CARTESIAN_POINT ( 'NONE',  ( 187.5000000000000000, 9.429780353434619030E-16, -7.700000000000000178 ) ) ;
#33606=CARTESIAN_POINT ( 'NONE',  ( 186.9166666666666856, 6.668395609140176816, 3.850000000000000977 ) ) ;
#33629=PLANE ( 'NONE',  #84093 ) ;
#33632=ORIENTED_EDGE ( 'NONE', *, *, #35070, .T. ) ;
#33653=CARTESIAN_POINT ( 'NONE',  ( 187.5000000000000000, 0.000000000000000000, 0.000000000000000000 ) ) ;
#33663=VERTEX_POINT ( 'NONE', #22856 ) ;
#33668=ORIENTED_EDGE ( 'NONE', *, *, #123557, .T. ) ;
#33699=ORIENTED_EDGE ( 'NONE', *, *, #126795, .T. ) ;
#33706=CARTESIAN_POINT ( 'NONE',  ( 129.5000000000000000, 0.000000000000000000, 0.000000000000000000 ) ) ;
#33774=DIRECTION ( 'NONE',  ( 0.000000000000000000, 0.000000000000000000, 1.000000000000000000 ) ) ;
#33838=CARTESIAN_POINT ( 'NONE',  ( 185.5312500006828031, 9.429780353434619030E-16, -7.700000000000000178 ) ) ;
#33886=CARTESIAN_POINT ( 'NONE',  ( 184.4010416670080872, -4.367472073101519747, 7.564683531249999149 ) ) ;
#33900=CARTESIAN_POINT ( 'NONE',  ( 179.5000000000000000, 1.375000000000000222, 6.000000000000000000 ) ) ;
#33929=ADVANCED_FACE ( 'NONE', ( #100576 ), #20743, .F. ) ;
#33949=ADVANCED_FACE ( 'NONE', ( #103169 ), #92050, .T. ) ;
#33999=CARTESIAN_POINT ( 'NONE',  ( 186.9479166673494603, -6.668395609140176816, -3.850000000000003642 ) ) ;
#34019=CARTESIAN_POINT ( 'NONE',  ( 103.0416120702864475, 7.673033776031224384, -0.6654386271658147001 ) ) ;
#34108=LINE ( 'NONE', #2688, #50186 ) ;
#34144=CARTESIAN_POINT ( 'NONE',  ( 127.5000000000000000, 1.500000000000000000, -6.000000000000000000 ) ) ;
#34152=ORIENTED_EDGE ( 'NONE', *, *, #116007, .F. ) ;
#34242=EDGE_CURVE ( 'NONE', #5682, #19872, #77869, .T. ) ;
#34260=CARTESIAN_POINT ( 'NONE',  ( 187.5000000000000000, 0.000000000000000000, 0.000000000000000000 ) ) ;
#34262=CARTESIAN_POINT ( 'NONE',  ( 185.4218750003414016, 0.000000000000000000, 7.564683531250000925 ) ) ;
#34267=CARTESIAN_POINT ( 'NONE',  ( 187.5000000000000000, 0.000000000000000000, 0.000000000000000000 ) ) ;
#34312=VECTOR ( 'NONE', #67712, 1000.000000000000000 ) ;
#34406=PLANE ( 'NONE',  #35336 ) ;
#34447=ORIENTED_EDGE ( 'NONE', *, *, #115661, .F. ) ;
#34473=ORIENTED_EDGE ( 'NONE', *, *, #245, .F. ) ;
#34511=CARTESIAN_POINT ( 'NONE',  ( 185.3645833340161175, -6.668395609140180369, 3.849999999999994760 ) ) ;
#34579=ORIENTED_EDGE ( 'NONE', *, *, #9429, .T. ) ;
#34590=TOROIDAL_SURFACE ( 'NONE', #1111, 8.199999999999999289, 0.5000000000000000000 ) ;
#34609=DIRECTION ( 'NONE',  ( 1.000000000000000000, 0.000000000000000000, 0.000000000000000000 ) ) ;
#34683=CARTESIAN_POINT ( 'NONE',  ( 106.3499248685753997, 6.077234604209151847, -4.730958255624227782 ) ) ;
#34793=ORIENTED_EDGE ( 'NONE', *, *, #50183, .F. ) ;
#34794=EDGE_CURVE ( 'NONE', #15661, #85617, #77691, .T. ) ;
#34876=ORIENTED_EDGE ( 'NONE', *, *, #110318, .T. ) ;
#34910=CARTESIAN_POINT ( 'NONE',  ( 184.2135416670080588, 4.367472073101518859, -7.564683531249999149 ) ) ;
#34971=ORIENTED_EDGE ( 'NONE', *, *, #71695, .T. ) ;
#34979=ADVANCED_FACE ( 'NONE', ( #26083 ), #115072, .F. ) ;
#35065=ORIENTED_EDGE ( 'NONE', *, *, #57081, .T. ) ;
#35070=EDGE_CURVE ( 'NONE', #16557, #33663, #88183, .T. ) ;
#35095=VECTOR ( 'NONE', #114057, 1000.000000000000000 ) ;
#35111=DIRECTION ( 'NONE',  ( -1.000000000000000000, 0.000000000000000000, 0.000000000000000000 ) ) ;
#35136=CARTESIAN_POINT ( 'NONE',  ( 186.8333333333333144, 6.668395609140177704, -3.849999999999998312 ) ) ;
#35142=AXIS2_PLACEMENT_3D ( 'NONE', #129039, #69435, #79283 ) ;
#35154=CARTESIAN_POINT ( 'NONE',  ( 184.0312500006828031, 9.429780353434619030E-16, -7.700000000000000178 ) ) ;
#35187=CYLINDRICAL_SURFACE ( 'NONE', #73038, 3.000000000000000444 ) ;
#35195=CARTESIAN_POINT ( 'NONE',  ( 185.2135416670080872, 4.367472073101518859, -7.564683531249999149 ) ) ;
#35262=FACE_OUTER_BOUND ( 'NONE', #88717, .T. ) ;
#35336=AXIS2_PLACEMENT_3D ( 'NONE', #16011, #16651, #45508 ) ;
#35407=ADVANCED_FACE ( 'NONE', ( #44254 ), #5608, .F. ) ;
#35467=LINE ( 'NONE', #16429, #40170 ) ;
#35502=AXIS2_PLACEMENT_3D ( 'NONE', #34260, #74171, #101699 ) ;
#35547=CARTESIAN_POINT ( 'NONE',  ( 187.4583333333333428, 4.445597072760117285, 7.699999999999999289 ) ) ;
#35646=ORIENTED_EDGE ( 'NONE', *, *, #92781, .F. ) ;
#35659=EDGE_CURVE ( 'NONE', #15804, #21810, #70353, .T. ) ;
#35765=VECTOR ( 'NONE', #78544, 1000.000000000000000 ) ;
#35781=CARTESIAN_POINT ( 'NONE',  ( 183.7812500006828031, 0.000000000000000000, 7.700000000000000178 ) ) ;
#35823=CARTESIAN_POINT ( 'NONE',  ( 184.3802083336747444, 4.367472073101515306, 7.564683531250000925 ) ) ;
#35892=CARTESIAN_POINT ( 'NONE',  ( 186.0468750003414300, -8.734944146203032389, -1.604583208406767949E-15 ) ) ;
#35992=ADVANCED_FACE ( 'NONE', ( #37530 ), #77438, .F. ) ;
#36113=FACE_OUTER_BOUND ( 'NONE', #49214, .T. ) ;
#36116=ORIENTED_EDGE ( 'NONE', *, *, #115661, .T. ) ;
#36194=CARTESIAN_POINT ( 'NONE',  ( 186.0000000000000000, 0.000000000000000000, 7.700000000000000178 ) ) ;
#36325=ORIENTED_EDGE ( 'NONE', *, *, #1698, .T. ) ;
#36446=CARTESIAN_POINT ( 'NONE',  ( 186.9843750003414300, -8.734944146203032389, -1.604583208406768146E-15 ) ) ;
#36489=CARTESIAN_POINT ( 'NONE',  ( 185.5052083336747444, -6.551208109652278289, 3.782341765624995134 ) ) ;
#36556=CARTESIAN_POINT ( 'NONE',  ( 184.9218750003414016, 0.000000000000000000, 7.564683531250000925 ) ) ;
#36586=EDGE_LOOP ( 'NONE', ( #78246, #36325 ) ) ;
#36681=EDGE_CURVE ( 'NONE', #109041, #118850, #64329, .T. ) ;
#36816=( BOUNDED_CURVE ( )  B_SPLINE_CURVE ( 2, ( #12495, #11847, #52421, #33449, #82545, #115849, #75924 ),
 .UNSPECIFIED., .F., .F. ) 
 B_SPLINE_CURVE_WITH_KNOTS ( ( 3, 2, 2, 3 ),
 ( 0.000000000000000000, 0.02380952380952383249, 0.04761904761904766498, 0.07142857142857149400 ),
 .UNSPECIFIED. ) 
 CURVE ( )  GEOMETRIC_REPRESENTATION_ITEM ( )  RATIONAL_B_SPLINE_CURVE ( ( 1.000000000000000000, 0.8660254037844387076, 1.000000000000000000, 0.8660254037844387076, 1.000000000000000000, 0.8660254037844383745, 1.000000000000000444 ) ) 
 REPRESENTATION_ITEM ( '' )  );
#36834=CARTESIAN_POINT ( 'NONE',  ( 186.5416666666666856, -4.445597072760122614, 7.699999999999998401 ) ) ;
#36862=CARTESIAN_POINT ( 'NONE',  ( 186.7500000000000000, 9.429780353434619030E-16, -7.700000000000000178 ) ) ;
#36919=ORIENTED_EDGE ( 'NONE', *, *, #72625, .F. ) ;
#37070=LINE ( 'NONE', #96597, #78001 ) ;
#37078=CARTESIAN_POINT ( 'NONE',  ( 184.2395833340161175, 4.445597072760117285, 7.699999999999999289 ) ) ;
#37104=VECTOR ( 'NONE', #60229, 1000.000000000000114 ) ;
#37122=CARTESIAN_POINT ( 'NONE',  ( 185.8385416670080872, 6.551208109652274736, 3.782341765625001351 ) ) ;
#37142=CIRCLE ( 'NONE', #110288, 7.700000000000000178 ) ;
#37174=DIRECTION ( 'NONE',  ( 0.000000000000000000, 0.000000000000000000, -1.000000000000000000 ) ) ;
#37194=CARTESIAN_POINT ( 'NONE',  ( 185.5052083336747444, -6.551208109652278289, 3.782341765624995134 ) ) ;
#37245=ORIENTED_EDGE ( 'NONE', *, *, #80456, .T. ) ;
#37247=DIRECTION ( 'NONE',  ( 1.000000000000000000, 0.000000000000000000, 0.000000000000000000 ) ) ;
#37257=ORIENTED_EDGE ( 'NONE', *, *, #62717, .T. ) ;
#37376=ADVANCED_FACE ( 'NONE', ( #104322 ), #123952, .F. ) ;
#37378=CARTESIAN_POINT ( 'NONE',  ( 129.5000000000000000, 1.500000000000000000, -2.598076211353316900 ) ) ;
#37417=( NAMED_UNIT ( * ) SI_UNIT ( $, .STERADIAN. ) SOLID_ANGLE_UNIT ( ) );
#37466=LINE ( 'NONE', #15864, #108692 ) ;
#37484=CARTESIAN_POINT ( 'NONE',  ( 186.3750000000000284, 8.891194145520236347, 5.444286225454521982E-16 ) ) ;
#37530=FACE_OUTER_BOUND ( 'NONE', #7161, .T. ) ;
#37586=( BOUNDED_SURFACE ( )  B_SPLINE_SURFACE ( 1, 2, ( 
 ( #61789, #80783, #12651, #59869, #89932, #110227, #31669, #1551, #89295, #110854, #71590, #99769, #111508, #129254, #120691, #120051, #40206, #61128, #10093, #50047, #21864, #101049, #11375, #82046, #256, #30405, #32341, #20563, #51332, #60503, #31049, #100411, #10707, #50662, #90577, #70947, #4759, #114094, #83356, #54512, #74815, #123904, #2847, #93814, #83972, #75444, #3495, #113446, #34262, #44720, #44063, #102977, #73512, #84634, #55176, #63060, #74172, #72884, #115351, #124567, #64975, #63710, #24423, #53885, #114730, #104898, #15221, #112811, #4119, #103637, #64345, #104274, #14584, #94438, #42808, #5416, #13946, #34910, #25066, #53249, #95103, #23787, #122629, #45367, #85271 ),
 ( #125204, #35547, #25707, #65629, #105565, #52590, #13296, #92513, #82719, #32975, #23132, #93181, #43441, #123271, #33606, #16515, #106831, #117278, #117946, #57101, #28950, #95745, #56449, #36834, #47941, #57763, #78700, #37484, #7994, #6053, #87839, #128449, #97029, #6680, #96365, #77393, #36194, #76103, #38116, #27623, #67549, #18467, #116019, #68854, #98305, #97671, #107498, #46009, #47296, #106211, #85903, #46643, #15882, #125832, #127775, #17812, #86558, #78035, #28295, #87197, #26368, #7344, #127149, #38784, #126496, #76748, #68204, #108134, #58413, #66277, #116663, #8625, #48583, #27009, #88490, #66909, #118596, #55815, #17140, #119895, #41984, #101545, #70789, #100883, #110705 ) ),
 .UNSPECIFIED., .F., .F., .F. ) 
 B_SPLINE_SURFACE_WITH_KNOTS ( ( 2, 2 ),
 ( 3, 2, 2, 2, 2, 2, 2, 2, 2, 2, 2, 2, 2, 2, 2, 2, 2, 2, 2, 2, 2, 2, 2, 2, 2, 2, 2, 2, 2, 2, 2, 2, 2, 2, 2, 2, 2, 2, 2, 2, 2, 2, 3 ),
 ( 0.000000000000000000, 1.000000000000000000 ),
 ( 0.000000000000000000, 0.02380952380952380820, 0.04761904761904761640, 0.07142857142857142461, 0.09523809523809523281, 0.1190476190476190410, 0.1428571428571428492, 0.1666666666666666574, 0.1904761904761904656, 0.2142857142857142738, 0.2380952380952380820, 0.2619047619047619180, 0.2857142857142856984, 0.3095238095238095344, 0.3333333333333333148, 0.3571428571428571508, 0.3809523809523809312, 0.4047619047619047672, 0.4285714285714285476, 0.4523809523809523836, 0.4761904761904761640, 0.5000000000000000000, 0.5238095238095238360, 0.5476190476190476719, 0.5714285714285713969, 0.5952380952380952328, 0.6190476190476190688, 0.6428571428571429047, 0.6666666666666666297, 0.6904761904761904656, 0.7142857142857143016, 0.7380952380952381375, 0.7619047619047618625, 0.7857142857142856984, 0.8095238095238095344, 0.8333333333333333703, 0.8571428571428570953, 0.8809523809523809312, 0.9047619047619047672, 0.9285714285714286031, 0.9523809523809523281, 0.9761904761904761640, 1.000000000000000000 ),
 .UNSPECIFIED. ) 
 GEOMETRIC_REPRESENTATION_ITEM ( )  RATIONAL_B_SPLINE_SURFACE ( (
 ( 1.000000000000000000, 0.8660254037844387076, 1.000000000000000000, 0.8660254037844387076, 1.000000000000000000, 0.8660254037844387076, 1.000000000000000000, 0.8660254037844387076, 1.000000000000000000, 0.8660254037844387076, 1.000000000000000000, 0.8660254037844387076, 1.000000000000000000, 0.8660254037844387076, 1.000000000000000000, 0.8660254037844387076, 1.000000000000000000, 0.8660254037844387076, 1.000000000000000000, 0.8660254037844387076, 1.000000000000000000, 0.8660254037844387076, 1.000000000000000000, 0.8660254037844387076, 1.000000000000000000, 0.8660254037844387076, 1.000000000000000000, 0.8660254037844387076, 1.000000000000000000, 0.8660254037844387076, 1.000000000000000000, 0.8660254037844387076, 1.000000000000000000, 0.8660254037844387076, 1.000000000000000000, 0.8660254037844387076, 1.000000000000000000, 0.8660254037844387076, 1.000000000000000000, 0.8660254037844387076, 1.000000000000000000, 0.8660254037844387076, 1.000000000000000000, 0.8660254037844387076, 1.000000000000000000, 0.8660254037844387076, 1.000000000000000000, 0.8660254037844387076, 1.000000000000000000, 0.8660254037844387076, 1.000000000000000000, 0.8660254037844387076, 1.000000000000000000, 0.8660254037844387076, 1.000000000000000000, 0.8660254037844387076, 1.000000000000000000, 0.8660254037844387076, 1.000000000000000000, 0.8660254037844387076, 1.000000000000000000, 0.8660254037844387076, 1.000000000000000000, 0.8660254037844387076, 1.000000000000000000, 0.8660254037844387076, 1.000000000000000000, 0.8660254037844387076, 1.000000000000000000, 0.8660254037844387076, 1.000000000000000000, 0.8660254037844387076, 1.000000000000000000, 0.8660254037844387076, 1.000000000000000000, 0.8660254037844387076, 1.000000000000000000, 0.8660254037844387076, 1.000000000000000000, 0.8660254037844387076, 1.000000000000000000, 0.8660254037844387076, 1.000000000000000000, 0.8660254037844387076, 1.000000000000000000),
 ( 1.000000000000000000, 0.8660254037844387076, 1.000000000000000000, 0.8660254037844387076, 1.000000000000000000, 0.8660254037844387076, 1.000000000000000000, 0.8660254037844387076, 1.000000000000000000, 0.8660254037844387076, 1.000000000000000000, 0.8660254037844387076, 1.000000000000000000, 0.8660254037844387076, 1.000000000000000000, 0.8660254037844387076, 1.000000000000000000, 0.8660254037844387076, 1.000000000000000000, 0.8660254037844387076, 1.000000000000000000, 0.8660254037844387076, 1.000000000000000000, 0.8660254037844387076, 1.000000000000000000, 0.8660254037844387076, 1.000000000000000000, 0.8660254037844387076, 1.000000000000000000, 0.8660254037844387076, 1.000000000000000000, 0.8660254037844387076, 1.000000000000000000, 0.8660254037844387076, 1.000000000000000000, 0.8660254037844387076, 1.000000000000000000, 0.8660254037844387076, 1.000000000000000000, 0.8660254037844387076, 1.000000000000000000, 0.8660254037844387076, 1.000000000000000000, 0.8660254037844387076, 1.000000000000000000, 0.8660254037844387076, 1.000000000000000000, 0.8660254037844387076, 1.000000000000000000, 0.8660254037844387076, 1.000000000000000000, 0.8660254037844387076, 1.000000000000000000, 0.8660254037844387076, 1.000000000000000000, 0.8660254037844387076, 1.000000000000000000, 0.8660254037844387076, 1.000000000000000000, 0.8660254037844387076, 1.000000000000000000, 0.8660254037844387076, 1.000000000000000000, 0.8660254037844387076, 1.000000000000000000, 0.8660254037844387076, 1.000000000000000000, 0.8660254037844387076, 1.000000000000000000, 0.8660254037844387076, 1.000000000000000000, 0.8660254037844387076, 1.000000000000000000, 0.8660254037844387076, 1.000000000000000000, 0.8660254037844387076, 1.000000000000000000, 0.8660254037844387076, 1.000000000000000000, 0.8660254037844387076, 1.000000000000000000, 0.8660254037844387076, 1.000000000000000000, 0.8660254037844387076, 1.000000000000000000) ) ) 
 REPRESENTATION_ITEM ( '' )  SURFACE ( )  );
#37666=EDGE_CURVE ( 'NONE', #48297, #125237, #94162, .T. ) ;
#37716=CARTESIAN_POINT ( 'NONE',  ( 184.2812500006828031, 0.000000000000000000, 7.700000000000000178 ) ) ;
#37798=ORIENTED_EDGE ( 'NONE', *, *, #68730, .T. ) ;
#37824=CARTESIAN_POINT ( 'NONE',  ( 185.1718750003414016, 9.264065473108010111E-16, -7.564683531250000925 ) ) ;
#37905=CARTESIAN_POINT ( 'NONE',  ( 186.4843750003414016, -8.734944146203032389, -1.604583208406768146E-15 ) ) ;
#37942=ADVANCED_FACE ( 'NONE', ( #8369 ), #48308, .F. ) ;
#37969=FACE_OUTER_BOUND ( 'NONE', #87337, .T. ) ;
#38025=DIRECTION ( 'NONE',  ( -1.000000000000000000, -0.000000000000000000, -0.000000000000000000 ) ) ;
#38116=CARTESIAN_POINT ( 'NONE',  ( 185.9166666666666856, 6.668395609140176816, 3.850000000000000977 ) ) ;
#38160=CARTESIAN_POINT ( 'NONE',  ( 187.2343750003414016, 8.734944146203032389, 5.348610694689227483E-16 ) ) ;
#38255=EDGE_CURVE ( 'NONE', #1392, #33034, #24653, .T. ) ;
#38278=CARTESIAN_POINT ( 'NONE',  ( 186.7500000000000000, 9.429780353434619030E-16, -7.700000000000000178 ) ) ;
#38305=DIRECTION ( 'NONE',  ( 0.000000000000000000, 0.000000000000000000, -1.000000000000000000 ) ) ;
#38350=( BOUNDED_CURVE ( )  B_SPLINE_CURVE ( 2, ( #16925, #76539, #26786, #77805, #66700, #96801, #126931 ),
 .UNSPECIFIED., .F., .F. ) 
 B_SPLINE_CURVE_WITH_KNOTS ( ( 3, 2, 2, 3 ),
 ( 0.07142857142857149400, 0.09523809523809532995, 0.1190476190476191520, 0.1428571428571429880 ),
 .UNSPECIFIED. ) 
 CURVE ( )  GEOMETRIC_REPRESENTATION_ITEM ( )  RATIONAL_B_SPLINE_CURVE ( ( 0.9999999999999996669, 0.8660254037844390407, 1.000000000000000000, 0.8660254037844387076, 1.000000000000000000, 0.8660254037844379305, 1.000000000000000666 ) ) 
 REPRESENTATION_ITEM ( '' )  );
#38367=ORIENTED_EDGE ( 'NONE', *, *, #2523, .T. ) ;
#38376=CARTESIAN_POINT ( 'NONE',  ( 185.1093750003413732, 9.264065473108010111E-16, -7.564683531250000925 ) ) ;
#38386=VERTEX_POINT ( 'NONE', #118182 ) ;
#38393=ORIENTED_EDGE ( 'NONE', *, *, #54408, .F. ) ;
#38412=PLANE ( 'NONE',  #7174 ) ;
#38446=CARTESIAN_POINT ( 'NONE',  ( 185.2500000000000000, 9.429780353434619030E-16, -7.700000000000000178 ) ) ;
#38459=AXIS2_PLACEMENT_3D ( 'NONE', #39479, #119289, #117323 ) ;
#38495=CARTESIAN_POINT ( 'NONE',  ( 184.1302083336747160, -4.367472073101514418, -7.564683531250002702 ) ) ;
#38580=CARTESIAN_POINT ( 'NONE',  ( 187.2343750003414016, 8.734944146203032389, 5.348610694689227483E-16 ) ) ;
#38619=LINE ( 'NONE', #117773, #35765 ) ;
#38655=CARTESIAN_POINT ( 'NONE',  ( 187.5000000000000000, 1.500000000000000000, 6.000000000000000000 ) ) ;
#38784=CARTESIAN_POINT ( 'NONE',  ( 184.8750000000000000, 8.891194145520236347, 5.444286225454521982E-16 ) ) ;
#38837=CARTESIAN_POINT ( 'NONE',  ( 104.6953598897069497, 7.846636665918518716, -3.765776865403877682 ) ) ;
#38856=DIRECTION ( 'NONE',  ( -1.000000000000000000, -0.000000000000000000, -0.000000000000000000 ) ) ;
#38894=ORIENTED_EDGE ( 'NONE', *, *, #1629, .F. ) ;
#38914=CARTESIAN_POINT ( 'NONE',  ( 112.8328331032861485, 8.604841203010149542, -1.324313734004374910 ) ) ;
#38933=CARTESIAN_POINT ( 'NONE',  ( 184.2395833340161460, 4.445597072760201662, 7.699999999999855405 ) ) ;
#38994=CARTESIAN_POINT ( 'NONE',  ( 129.5000000000000000, -0.6250000000000028866, -7.634788798650553154 ) ) ;
#39035=CARTESIAN_POINT ( 'NONE',  ( 184.6927083336747160, 6.551208109652275624, -3.782341765624998686 ) ) ;
#39189=DIRECTION ( 'NONE',  ( 0.000000000000000000, 0.000000000000000000, -1.000000000000000000 ) ) ;
#39205=CARTESIAN_POINT ( 'NONE',  ( 129.5000000000000000, -1.375000000000000000, 7.576237522675751457 ) ) ;
#39233=VERTEX_POINT ( 'NONE', #115265 ) ;
#39235=CARTESIAN_POINT ( 'NONE',  ( 186.6093750003414016, 9.264065473108010111E-16, -7.564683531250000925 ) ) ;
#39310=FACE_OUTER_BOUND ( 'NONE', #36586, .T. ) ;
#39324=EDGE_LOOP ( 'NONE', ( #12637, #68582, #70641, #117750 ) ) ;
#39327=ADVANCED_FACE ( 'NONE', ( #75362 ), #25615, .F. ) ;
#39332=CARTESIAN_POINT ( 'NONE',  ( 184.6979166673494603, 6.668395609140176816, 3.850000000000000977 ) ) ;
#39335=VECTOR ( 'NONE', #10329, 1000.000000000000000 ) ;
#39350=DIRECTION ( 'NONE',  ( -1.000000000000000000, -0.000000000000000000, -0.000000000000000000 ) ) ;
#39431=LINE ( 'NONE', #32185, #118494 ) ;
#39441=ORIENTED_EDGE ( 'NONE', *, *, #126703, .T. ) ;
#39474=CARTESIAN_POINT ( 'NONE',  ( 186.6093750003414016, 9.264065473108010111E-16, -7.564683531250000925 ) ) ;
#39479=CARTESIAN_POINT ( 'NONE',  ( 108.0000000000000142, 8.700999999999998735, 0.000000000000000000 ) ) ;
#39518=CARTESIAN_POINT ( 'NONE',  ( 185.1666666666666856, -6.668395609140176816, -3.850000000000003642 ) ) ;
#39546=AXIS2_PLACEMENT_3D ( 'NONE', #50991, #12329, #100704 ) ;
#39570=CARTESIAN_POINT ( 'NONE',  ( 129.5000000000000000, 0.000000000000000000, 0.000000000000000000 ) ) ;
#39577=CARTESIAN_POINT ( 'NONE',  ( 184.1562500006828031, 8.891194145520236347, 5.444286225454521982E-16 ) ) ;
#39681=AXIS2_PLACEMENT_3D ( 'NONE', #22007, #30541, #101836 ) ;
#39720=ORIENTED_EDGE ( 'NONE', *, *, #99658, .T. ) ;
#39742=EDGE_CURVE ( 'NONE', #51279, #41599, #1630, .T. ) ;
#39747=EDGE_CURVE ( 'NONE', #59105, #2046, #118671, .T. ) ;
#39832=DIRECTION ( 'NONE',  ( 1.000000000000000000, 0.000000000000000000, 0.000000000000000000 ) ) ;
#39950=CARTESIAN_POINT ( 'NONE',  ( 185.7395833340161175, 4.445597072760159030, 7.699999999999928235 ) ) ;
#39984=CARTESIAN_POINT ( 'NONE',  ( 104.0450469811252532, 7.064712996401804723, 3.075733052666039580 ) ) ;
#40001=CARTESIAN_POINT ( 'NONE',  ( 185.7500000000000000, 9.429780353434619030E-16, -7.700000000000000178 ) ) ;
#40076=CARTESIAN_POINT ( 'NONE',  ( 185.4062500006828031, -8.891194145520236347, -1.633285867636356299E-15 ) ) ;
#40095=CARTESIAN_POINT ( 'NONE',  ( 187.0260416670080588, -6.551208109652273848, -3.782341765625003571 ) ) ;
#40170=VECTOR ( 'NONE', #115947, 1000.000000000000000 ) ;
#40178=CARTESIAN_POINT ( 'NONE',  ( 112.9918852365773603, 8.695328135426091620, 0.3304444235703573596 ) ) ;
#40206=CARTESIAN_POINT ( 'NONE',  ( 186.7552083336747444, 6.551208109652275624, -3.782341765624998686 ) ) ;
#40234=AXIS2_PLACEMENT_3D ( 'NONE', #61784, #72249, #44715 ) ;
#40238=CARTESIAN_POINT ( 'NONE',  ( 183.9062500006828031, -8.891194145520236347, -1.633285867636356299E-15 ) ) ;
#40301=CARTESIAN_POINT ( 'NONE',  ( 184.7343750003414016, 8.734944146203032389, 5.348610694689227483E-16 ) ) ;
#40333=ORIENTED_EDGE ( 'NONE', *, *, #43516, .T. ) ;
#40341=COLOUR_RGB ( '', 0.40784314, 0.44705882, 0.49803922) ;
#40503=CARTESIAN_POINT ( 'NONE',  ( 185.6666666666666856, -6.668395609140176816, -3.850000000000003642 ) ) ;
#40513=CARTESIAN_POINT ( 'NONE',  ( 186.4427083336747160, -6.551208109652278289, 3.782341765624995134 ) ) ;
#40576=EDGE_CURVE ( 'NONE', #100714, #39233, #86088, .T. ) ;
#40638=CARTESIAN_POINT ( 'NONE',  ( 129.5000000000000000, 0.000000000000000000, 6.000000000000000000 ) ) ;
#40696=ORIENTED_EDGE ( 'NONE', *, *, #26079, .T. ) ;
#40764=CARTESIAN_POINT ( 'NONE',  ( 106.3580756688206321, 7.300875089796112327, -4.733840378913477309 ) ) ;
#40787=CARTESIAN_POINT ( 'NONE',  ( 184.4062500006827747, -8.891194145520236347, -1.633285867636356299E-15 ) ) ;
#40837=CARTESIAN_POINT ( 'NONE',  ( 111.7562837278403549, 8.047280753376885087, 3.315426444331004863 ) ) ;
#40841=EDGE_CURVE ( 'NONE', #4435, #9738, #41932, .T. ) ;
#40872=FACE_OUTER_BOUND ( 'NONE', #121413, .T. ) ;
#40962=CARTESIAN_POINT ( 'NONE',  ( 184.8593750003413732, 0.000000000000000000, 7.564683531250000925 ) ) ;
#41051=DIRECTION ( 'NONE',  ( 1.000000000000000000, 0.000000000000000000, -0.000000000000000000 ) ) ;
#41084=LINE ( 'NONE', #71157, #25421 ) ;
#41156=CARTESIAN_POINT ( 'NONE',  ( 187.2552083336747444, 6.551208109652275624, -3.782341765624998686 ) ) ;
#41162=CARTESIAN_POINT ( 'NONE',  ( 179.5000000000000000, -0.6250000000000000000, 7.634788798650553154 ) ) ;
#41398=CARTESIAN_POINT ( 'NONE',  ( 185.1093750003413732, 9.264065473108010111E-16, -7.564683531250000925 ) ) ;
#41421=LINE ( 'NONE', #89846, #24972 ) ;
#41478=CARTESIAN_POINT ( 'NONE',  ( 187.5000000000000000, 1.500000000000000000, 6.000000000000000000 ) ) ;
#41522=FACE_OUTER_BOUND ( 'NONE', #6760, .T. ) ;
#41599=VERTEX_POINT ( 'NONE', #61814 ) ;
#41692=CARTESIAN_POINT ( 'NONE',  ( 186.3229166673494319, -4.445597072760092416, 7.700000000000049916 ) ) ;
#41752=CARTESIAN_POINT ( 'NONE',  ( 185.9895833340161460, -4.445597072760115509, -7.700000000000001954 ) ) ;
#41802=CARTESIAN_POINT ( 'NONE',  ( 184.5260416670080588, -6.551208109652273848, -3.782341765625003571 ) ) ;
#41910=CARTESIAN_POINT ( 'NONE',  ( 187.5000000000000000, 9.429780353434619030E-16, -7.700000000000000178 ) ) ;
#41915=ORIENTED_EDGE ( 'NONE', *, *, #73107, .T. ) ;
#41918=CARTESIAN_POINT ( 'NONE',  ( 105.7538778652931626, 6.265388825864785183, -4.478799985686444884 ) ) ;
#41932=LINE ( 'NONE', #51745, #111321 ) ;
#41960=DIRECTION ( 'NONE',  ( -1.000000000000000000, -0.000000000000000000, -0.000000000000000000 ) ) ;
#41984=CARTESIAN_POINT ( 'NONE',  ( 184.1666666666666856, -6.668395609140176816, -3.850000000000003642 ) ) ;
#42026=CARTESIAN_POINT ( 'NONE',  ( 184.3593750003413732, 0.000000000000000000, 7.564683531250000925 ) ) ;
#42039=ORIENTED_EDGE ( 'NONE', *, *, #47858, .F. ) ;
#42058=DIRECTION ( 'NONE',  ( 0.000000000000000000, 0.000000000000000000, -1.000000000000000000 ) ) ;
#42229=FACE_OUTER_BOUND ( 'NONE', #118154, .T. ) ;
#42242=ORIENTED_EDGE ( 'NONE', *, *, #18769, .T. ) ;
#42275=ORIENTED_EDGE ( 'NONE', *, *, #28022, .T. ) ;
#42290=ADVANCED_FACE ( 'NONE', ( #28167 ), #18334, .F. ) ;
#42321=CARTESIAN_POINT ( 'NONE',  ( 186.3645833340161175, -6.668395609140180369, 3.849999999999994760 ) ) ;
#42383=CARTESIAN_POINT ( 'NONE',  ( 185.8229166673494319, -4.445597072760122614, 7.699999999999998401 ) ) ;
#42405=CARTESIAN_POINT ( 'NONE',  ( 179.5000000000000000, -1.375000000000000000, 7.634788798650553154 ) ) ;
#42434=CARTESIAN_POINT ( 'NONE',  ( 187.1302083336747444, -4.367472073101514418, -7.564683531250002702 ) ) ;
#42511=CARTESIAN_POINT ( 'NONE',  ( 184.1666666666666856, -6.668395609140176816, -3.850000000000003642 ) ) ;
#42563=( BOUNDED_CURVE ( )  B_SPLINE_CURVE ( 2, ( #13600, #110046, #20378, #91046, #64006, #30856, #44358 ),
 .UNSPECIFIED., .F., .T. ) 
 B_SPLINE_CURVE_WITH_KNOTS ( ( 3, 2, 2, 3 ),
 ( 0.2857142857142859760, 0.3095238095238098119, 0.3333333333333335924, 0.3571428571428574283 ),
 .UNSPECIFIED. ) 
 CURVE ( )  GEOMETRIC_REPRESENTATION_ITEM ( )  RATIONAL_B_SPLINE_CURVE ( ( 0.9999999999999984457, 0.8660254037844402619, 1.000000000000000000, 0.8660254037844387076, 1.000000000000000000, 0.8660254037844371533, 1.000000000000001554 ) ) 
 REPRESENTATION_ITEM ( '' )  );
#42603=CARTESIAN_POINT ( 'NONE',  ( 185.9895833340161175, -4.445597072760145707, -7.699999999999951328 ) ) ;
#42622=EDGE_CURVE ( 'NONE', #99145, #93739, #81892, .T. ) ;
#42695=CARTESIAN_POINT ( 'NONE',  ( 185.0677083336747160, -4.367472073101514418, -7.564683531250002702 ) ) ;
#42760=CARTESIAN_POINT ( 'NONE',  ( 185.1562500006828031, 8.891194145520236347, 5.444286225454521982E-16 ) ) ;
#42765=SURFACE_SIDE_STYLE ('',( #23094 ) ) ;
#42791=DIRECTION ( 'NONE',  ( 0.000000000000000000, 0.000000000000000000, -1.000000000000000000 ) ) ;
#42804=EDGE_CURVE ( 'NONE', #64073, #59105, #48788, .T. ) ;
#42808=CARTESIAN_POINT ( 'NONE',  ( 184.3385416670080872, 6.551208109652274736, 3.782341765625001351 ) ) ;
#42829=VECTOR ( 'NONE', #49711, 1000.000000000000000 ) ;
#42895=ORIENTED_EDGE ( 'NONE', *, *, #50076, .T. ) ;
#42898=CARTESIAN_POINT ( 'NONE',  ( 185.7812500006828031, 0.000000000000000000, 7.700000000000000178 ) ) ;
#42940=ORIENTED_EDGE ( 'NONE', *, *, #37666, .T. ) ;
#43051=CARTESIAN_POINT ( 'NONE',  ( 186.2812500006828031, 0.000000000000000000, 7.700000000000000178 ) ) ;
#43096=CARTESIAN_POINT ( 'NONE',  ( 184.3593750003413732, 0.000000000000000000, 7.564683531250000925 ) ) ;
#43162=CARTESIAN_POINT ( 'NONE',  ( 184.2083333333333144, -4.445597072760187451, -7.699999999999876721 ) ) ;
#43167=VERTEX_POINT ( 'NONE', #108813 ) ;
#43216=CARTESIAN_POINT ( 'NONE',  ( 105.4682043743740110, 6.375218138983957061, -4.323317965031781007 ) ) ;
#43250=EDGE_CURVE ( 'NONE', #94263, #86875, #65074, .T. ) ;
#43268=VERTEX_POINT ( 'NONE', #34144 ) ;
#43323=( BOUNDED_CURVE ( )  B_SPLINE_CURVE ( 2, ( #129532, #9730, #40503, #60765, #120331, #25329, #44332 ),
 .UNSPECIFIED., .F., .F. ) 
 B_SPLINE_CURVE_WITH_KNOTS ( ( 3, 2, 2, 3 ),
 ( 0.5000000000000004441, 0.5238095238095242800, 0.5476190476190482270, 0.5714285714285719520 ),
 .UNSPECIFIED. ) 
 CURVE ( )  GEOMETRIC_REPRESENTATION_ITEM ( )  RATIONAL_B_SPLINE_CURVE ( ( 0.9999999999999974465, 0.8660254037844412611, 1.000000000000000000, 0.8660254037844387076, 1.000000000000000000, 0.8660254037844355990, 1.000000000000003109 ) ) 
 REPRESENTATION_ITEM ( '' )  );
#43328=CARTESIAN_POINT ( 'NONE',  ( 186.0677083336747444, -4.367472073101514418, -7.564683531250002702 ) ) ;
#43347=EDGE_CURVE ( 'NONE', #109625, #73015, #53514, .T. ) ;
#43361=CARTESIAN_POINT ( 'NONE',  ( 187.5000000000000000, 9.429780353434619030E-16, -7.700000000000000178 ) ) ;
#43441=CARTESIAN_POINT ( 'NONE',  ( 187.0000000000000000, 0.000000000000000000, 7.700000000000000178 ) ) ;
#43462=CARTESIAN_POINT ( 'NONE',  ( 129.5000000000000000, 0.000000000000000000, 0.000000000000000000 ) ) ;
#43516=EDGE_CURVE ( 'NONE', #79091, #73015, #97562, .T. ) ;
#43519=ADVANCED_FACE ( 'NONE', ( #98204 ), #109973, .F. ) ;
#43595=EDGE_CURVE ( 'NONE', #59835, #12583, #126257, .T. ) ;
#43691=CARTESIAN_POINT ( 'NONE',  ( 185.6562500006828316, 8.891194145520236347, 5.444286225454521982E-16 ) ) ;
#43735=CARTESIAN_POINT ( 'NONE',  ( 183.9010416670080588, -4.367472073101519747, 7.564683531249999149 ) ) ;
#43858=CARTESIAN_POINT ( 'NONE',  ( 103.1680366585140405, 7.591785779721488936, -1.328661963585094918 ) ) ;
#43861=ORIENTED_EDGE ( 'NONE', *, *, #126584, .T. ) ;
#43965=CARTESIAN_POINT ( 'NONE',  ( 185.9843750003414016, -8.734944146203032389, -1.604583208406767949E-15 ) ) ;
#44057=CARTESIAN_POINT ( 'NONE',  ( 187.4609375001707008, 0.000000000000000000, 7.632341765625000107 ) ) ;
#44063=CARTESIAN_POINT ( 'NONE',  ( 185.3385416670080872, 6.551208109652274736, 3.782341765625001351 ) ) ;
#44144=ORIENTED_EDGE ( 'NONE', *, *, #72496, .T. ) ;
#44167=DIRECTION ( 'NONE',  ( 1.000000000000000000, 0.000000000000000000, 0.000000000000000000 ) ) ;
#44206=ADVANCED_FACE ( 'NONE', ( #124791 ), #61919, .T. ) ;
#44254=FACE_OUTER_BOUND ( 'NONE', #82646, .T. ) ;
#44300=CARTESIAN_POINT ( 'NONE',  ( 185.4062500006828316, -8.891194145520236347, -1.633285867636356693E-15 ) ) ;
#44332=CARTESIAN_POINT ( 'NONE',  ( 185.5000000000000000, 0.000000000000000000, 7.700000000000000178 ) ) ;
#44345=CARTESIAN_POINT ( 'NONE',  ( 183.9635416670080872, -4.367472073101519747, 7.564683531249999149 ) ) ;
#44358=CARTESIAN_POINT ( 'NONE',  ( 186.2500000000000000, 9.429780353434619030E-16, -7.700000000000000178 ) ) ;
#44418=CARTESIAN_POINT ( 'NONE',  ( 187.2968750003414300, 8.734944146203032389, 5.348610694689227483E-16 ) ) ;
#44420=LINE ( 'NONE', #111208, #13477 ) ;
#44439=( BOUNDED_SURFACE ( )  B_SPLINE_SURFACE ( 1, 2, ( 
 ( #3732, #51564, #23360, #53495, #91470, #102571, #71845, #113042, #83599, #12255, #74418, #111764, #12887, #52196, #93410, #122238, #101305, #123501, #103234, #72493, #121565, #52840, #13547, #31917, #43051, #4350, #92775, #73751, #3105, #124153, #54130, #41752, #2428, #22116, #62024, #42383, #63952, #122877, #94055, #43691, #103877, #33221, #33838, #113699, #14183, #44300, #34511, #15477, #65876, #14815, #104510, #6289, #75685, #54756, #126744, #27236, #94688, #55422, #16108, #85520, #114963, #46895, #64585, #26604, #84873, #76355, #125444, #56680, #46237, #107078, #86139, #106447, #37716, #37078, #116895, #124809, #56046, #117528, #35154, #97272, #116259, #75060, #25290, #67138, #35781 ),
 ( #77621, #95346, #25965, #17402, #65219, #6928, #105149, #16754, #7596, #36446, #5012, #44964, #5652, #96607, #95990, #45613, #105809, #126079, #86805, #76990, #115610, #66513, #57350, #47539, #87441, #127388, #9548, #109681, #67809, #78299, #88067, #60596, #98540, #119482, #69747, #128025, #118204, #10795, #20015, #10189, #90014, #59962, #68447, #99864, #28541, #50128, #50758, #58008, #108380, #80223, #79576, #18709, #29829, #8875, #38376, #97911, #70396, #89393, #346, #78941, #40962, #128706, #109010, #40301, #39035, #58650, #48835, #69094, #120143, #88746, #118845, #29202, #20658, #30495, #110319, #19343, #59308, #90674, #100491, #48177, #99219, #1007, #80868, #18058, #49487 ) ),
 .UNSPECIFIED., .F., .F., .F. ) 
 B_SPLINE_SURFACE_WITH_KNOTS ( ( 2, 2 ),
 ( 3, 2, 2, 2, 2, 2, 2, 2, 2, 2, 2, 2, 2, 2, 2, 2, 2, 2, 2, 2, 2, 2, 2, 2, 2, 2, 2, 2, 2, 2, 2, 2, 2, 2, 2, 2, 2, 2, 2, 2, 2, 2, 3 ),
 ( 0.000000000000000000, 1.000000000000000000 ),
 ( 0.000000000000000000, 0.02380952380952380820, 0.04761904761904761640, 0.07142857142857142461, 0.09523809523809523281, 0.1190476190476190410, 0.1428571428571428492, 0.1666666666666666574, 0.1904761904761904656, 0.2142857142857142738, 0.2380952380952380820, 0.2619047619047619180, 0.2857142857142856984, 0.3095238095238095344, 0.3333333333333333148, 0.3571428571428571508, 0.3809523809523809312, 0.4047619047619047672, 0.4285714285714285476, 0.4523809523809523836, 0.4761904761904761640, 0.5000000000000000000, 0.5238095238095238360, 0.5476190476190476719, 0.5714285714285713969, 0.5952380952380952328, 0.6190476190476190688, 0.6428571428571429047, 0.6666666666666666297, 0.6904761904761904656, 0.7142857142857143016, 0.7380952380952381375, 0.7619047619047618625, 0.7857142857142856984, 0.8095238095238095344, 0.8333333333333333703, 0.8571428571428570953, 0.8809523809523809312, 0.9047619047619047672, 0.9285714285714286031, 0.9523809523809523281, 0.9761904761904761640, 1.000000000000000000 ),
 .UNSPECIFIED. ) 
 GEOMETRIC_REPRESENTATION_ITEM ( )  RATIONAL_B_SPLINE_SURFACE ( (
 ( 1.000000000000000000, 0.8660254037844387076, 1.000000000000000000, 0.8660254037844387076, 1.000000000000000000, 0.8660254037844387076, 1.000000000000000000, 0.8660254037844387076, 1.000000000000000000, 0.8660254037844387076, 1.000000000000000000, 0.8660254037844387076, 1.000000000000000000, 0.8660254037844387076, 1.000000000000000000, 0.8660254037844387076, 1.000000000000000000, 0.8660254037844387076, 1.000000000000000000, 0.8660254037844387076, 1.000000000000000000, 0.8660254037844387076, 1.000000000000000000, 0.8660254037844387076, 1.000000000000000000, 0.8660254037844387076, 1.000000000000000000, 0.8660254037844387076, 1.000000000000000000, 0.8660254037844387076, 1.000000000000000000, 0.8660254037844387076, 1.000000000000000000, 0.8660254037844387076, 1.000000000000000000, 0.8660254037844387076, 1.000000000000000000, 0.8660254037844387076, 1.000000000000000000, 0.8660254037844387076, 1.000000000000000000, 0.8660254037844387076, 1.000000000000000000, 0.8660254037844387076, 1.000000000000000000, 0.8660254037844387076, 1.000000000000000000, 0.8660254037844387076, 1.000000000000000000, 0.8660254037844387076, 1.000000000000000000, 0.8660254037844387076, 1.000000000000000000, 0.8660254037844387076, 1.000000000000000000, 0.8660254037844387076, 1.000000000000000000, 0.8660254037844387076, 1.000000000000000000, 0.8660254037844387076, 1.000000000000000000, 0.8660254037844387076, 1.000000000000000000, 0.8660254037844387076, 1.000000000000000000, 0.8660254037844387076, 1.000000000000000000, 0.8660254037844387076, 1.000000000000000000, 0.8660254037844387076, 1.000000000000000000, 0.8660254037844387076, 1.000000000000000000, 0.8660254037844387076, 1.000000000000000000, 0.8660254037844387076, 1.000000000000000000, 0.8660254037844387076, 1.000000000000000000, 0.8660254037844387076, 1.000000000000000000, 0.8660254037844387076, 1.000000000000000000, 0.8660254037844387076, 1.000000000000000000),
 ( 1.000000000000000000, 0.8660254037844387076, 1.000000000000000000, 0.8660254037844387076, 1.000000000000000000, 0.8660254037844387076, 1.000000000000000000, 0.8660254037844387076, 1.000000000000000000, 0.8660254037844387076, 1.000000000000000000, 0.8660254037844387076, 1.000000000000000000, 0.8660254037844387076, 1.000000000000000000, 0.8660254037844387076, 1.000000000000000000, 0.8660254037844387076, 1.000000000000000000, 0.8660254037844387076, 1.000000000000000000, 0.8660254037844387076, 1.000000000000000000, 0.8660254037844387076, 1.000000000000000000, 0.8660254037844387076, 1.000000000000000000, 0.8660254037844387076, 1.000000000000000000, 0.8660254037844387076, 1.000000000000000000, 0.8660254037844387076, 1.000000000000000000, 0.8660254037844387076, 1.000000000000000000, 0.8660254037844387076, 1.000000000000000000, 0.8660254037844387076, 1.000000000000000000, 0.8660254037844387076, 1.000000000000000000, 0.8660254037844387076, 1.000000000000000000, 0.8660254037844387076, 1.000000000000000000, 0.8660254037844387076, 1.000000000000000000, 0.8660254037844387076, 1.000000000000000000, 0.8660254037844387076, 1.000000000000000000, 0.8660254037844387076, 1.000000000000000000, 0.8660254037844387076, 1.000000000000000000, 0.8660254037844387076, 1.000000000000000000, 0.8660254037844387076, 1.000000000000000000, 0.8660254037844387076, 1.000000000000000000, 0.8660254037844387076, 1.000000000000000000, 0.8660254037844387076, 1.000000000000000000, 0.8660254037844387076, 1.000000000000000000, 0.8660254037844387076, 1.000000000000000000, 0.8660254037844387076, 1.000000000000000000, 0.8660254037844387076, 1.000000000000000000, 0.8660254037844387076, 1.000000000000000000, 0.8660254037844387076, 1.000000000000000000, 0.8660254037844387076, 1.000000000000000000, 0.8660254037844387076, 1.000000000000000000, 0.8660254037844387076, 1.000000000000000000, 0.8660254037844387076, 1.000000000000000000) ) ) 
 REPRESENTATION_ITEM ( '' )  SURFACE ( )  );
#44476=CARTESIAN_POINT ( 'NONE',  ( 107.6591838055444441, 5.855766388782936538, -5.000000000000004441 ) ) ;
#44506=LINE ( 'NONE', #15016, #48366 ) ;
#44542=VECTOR ( 'NONE', #127576, 1000.000000000000000 ) ;
#44559=CYLINDRICAL_SURFACE ( 'NONE', #100578, 7.700000000000000178 ) ;
#44715=DIRECTION ( 'NONE',  ( 0.000000000000000000, 0.000000000000000000, 1.000000000000000000 ) ) ;
#44718=ADVANCED_FACE ( 'NONE', ( #70064 ), #50416, .T. ) ;
#44720=CARTESIAN_POINT ( 'NONE',  ( 185.3802083336747160, 4.367472073101515306, 7.564683531250000925 ) ) ;
#44826=DIRECTION ( 'NONE',  ( -1.000000000000000000, 0.000000000000000000, 0.000000000000000000 ) ) ;
#44895=DIRECTION ( 'NONE',  ( 0.000000000000000000, -1.000000000000000000, 0.000000000000000000 ) ) ;
#44902=VERTEX_POINT ( 'NONE', #32090 ) ;
#44943=CARTESIAN_POINT ( 'NONE',  ( 187.0000000000000000, 0.000000000000000000, 7.700000000000000178 ) ) ;
#44964=CARTESIAN_POINT ( 'NONE',  ( 186.9010416670080303, -4.367472073101519747, 7.564683531249999149 ) ) ;
#45000=CARTESIAN_POINT ( 'NONE',  ( 184.0000000000000000, 0.000000000000000000, 7.700000000000000178 ) ) ;
#45009=CARTESIAN_POINT ( 'NONE',  ( 185.2968750003414300, 8.734944146203032389, 5.348610694689227483E-16 ) ) ;
#45053=FACE_OUTER_BOUND ( 'NONE', #24559, .T. ) ;
#45213=VECTOR ( 'NONE', #117867, 1000.000000000000000 ) ;
#45219=CARTESIAN_POINT ( 'NONE',  ( 129.5000000000000000, -1.000000000000025535, 7.634788798650553154 ) ) ;
#45248=ORIENTED_EDGE ( 'NONE', *, *, #6678, .T. ) ;
#45322=DIRECTION ( 'NONE',  ( -1.000000000000000000, 0.000000000000000000, -0.000000000000000000 ) ) ;
#45367=CARTESIAN_POINT ( 'NONE',  ( 183.9635416670080872, -4.367472073101519747, 7.564683531249999149 ) ) ;
#45508=DIRECTION ( 'NONE',  ( 0.000000000000000000, 1.846105847067148761E-16, 1.000000000000000000 ) ) ;
#45515=CARTESIAN_POINT ( 'NONE',  ( 179.5000000000000000, 0.000000000000000000, 0.000000000000000000 ) ) ;
#45613=CARTESIAN_POINT ( 'NONE',  ( 186.7343750003414300, 8.734944146203032389, 5.348610694689227483E-16 ) ) ;
#45655=CARTESIAN_POINT ( 'NONE',  ( 184.0885416670080872, -6.551208109652273848, -3.782341765625003571 ) ) ;
#45722=CARTESIAN_POINT ( 'NONE',  ( 185.3385416670080872, 6.551208109652274736, 3.782341765625001351 ) ) ;
#45792=CARTESIAN_POINT ( 'NONE',  ( 187.5000000000000000, -1.000000000000025535, 7.634788798650553154 ) ) ;
#45844=EDGE_CURVE ( 'NONE', #14892, #86875, #89156, .T. ) ;
#45896=DIRECTION ( 'NONE',  ( 0.000000000000000000, 1.224646799147353454E-16, 1.000000000000000000 ) ) ;
#45951=CARTESIAN_POINT ( 'NONE',  ( 87.50000000000001421, 0.000000000000000000, 0.000000000000000000 ) ) ;
#45992=( BOUNDED_CURVE ( )  B_SPLINE_CURVE ( 2, ( #31625, #101657, #11968, #42760, #82667, #122582, #15832 ),
 .UNSPECIFIED., .F., .F. ) 
 B_SPLINE_CURVE_WITH_KNOTS ( ( 3, 2, 2, 3 ),
 ( 0.5714285714285719520, 0.5952380952380957879, 0.6190476190476195129, 0.6428571428571433488 ),
 .UNSPECIFIED. ) 
 CURVE ( )  GEOMETRIC_REPRESENTATION_ITEM ( )  RATIONAL_B_SPLINE_CURVE ( ( 0.9999999999999968914, 0.8660254037844418162, 1.000000000000000000, 0.8660254037844387076, 1.000000000000000000, 0.8660254037844361541, 1.000000000000002442 ) ) 
 REPRESENTATION_ITEM ( '' )  );
#46009=CARTESIAN_POINT ( 'NONE',  ( 185.5416666666666572, -4.445597072760122614, 7.699999999999998401 ) ) ;
#46116=ORIENTED_EDGE ( 'NONE', *, *, #127473, .F. ) ;
#46166=ORIENTED_EDGE ( 'NONE', *, *, #34242, .T. ) ;
#46167=CYLINDRICAL_SURFACE ( 'NONE', #90458, 7.700000000000000178 ) ;
#46204=ORIENTED_EDGE ( 'NONE', *, *, #21838, .T. ) ;
#46237=CARTESIAN_POINT ( 'NONE',  ( 184.4479166673494603, -6.668395609140176816, -3.850000000000003642 ) ) ;
#46253=ORIENTED_EDGE ( 'NONE', *, *, #64591, .T. ) ;
#46277=CARTESIAN_POINT ( 'NONE',  ( 185.9635416670080872, -4.367472073101519747, 7.564683531249999149 ) ) ;
#46344=CARTESIAN_POINT ( 'NONE',  ( 185.9218750003414016, 0.000000000000000000, 7.564683531250000925 ) ) ;
#46349=ORIENTED_EDGE ( 'NONE', *, *, #15719, .F. ) ;
#46423=ORIENTED_EDGE ( 'NONE', *, *, #7166, .T. ) ;
#46453=CARTESIAN_POINT ( 'NONE',  ( 129.5000000000000000, -1.375000000000000222, 6.000000000000000000 ) ) ;
#46527=AXIS2_PLACEMENT_3D ( 'NONE', #45515, #76894, #55954 ) ;
#46588=EDGE_CURVE ( 'NONE', #128722, #15804, #63882, .T. ) ;
#46643=CARTESIAN_POINT ( 'NONE',  ( 185.3750000000000284, 8.891194145520236347, 5.444286225454521982E-16 ) ) ;
#46677=CARTESIAN_POINT ( 'NONE',  ( 129.5000000000000000, 1.375000000000002665, -7.576237522675752345 ) ) ;
#46753=( BOUNDED_CURVE ( )  B_SPLINE_CURVE ( 2, ( #2635, #42603, #63520, #23579, #103442, #13746, #93615 ),
 .UNSPECIFIED., .F., .F. ) 
 B_SPLINE_CURVE_WITH_KNOTS ( ( 3, 2, 2, 3 ),
 ( 0.3571428571428574283, 0.3809523809523812643, 0.4047619047619051003, 0.4285714285714289362 ),
 .UNSPECIFIED. ) 
 CURVE ( )  GEOMETRIC_REPRESENTATION_ITEM ( )  RATIONAL_B_SPLINE_CURVE ( ( 0.9999999999999984457, 0.8660254037844402619, 1.000000000000000000, 0.8660254037844387076, 1.000000000000000000, 0.8660254037844364872, 1.000000000000002220 ) ) 
 REPRESENTATION_ITEM ( '' )  );
#46775=ORIENTED_EDGE ( 'NONE', *, *, #13713, .T. ) ;
#46828=CARTESIAN_POINT ( 'NONE',  ( 185.2812500006828031, 0.000000000000000000, 7.700000000000000178 ) ) ;
#46882=AXIS2_PLACEMENT_3D ( 'NONE', #38655, #49111, #19639 ) ;
#46895=CARTESIAN_POINT ( 'NONE',  ( 184.7395833340161460, 4.445597072760117285, 7.699999999999999289 ) ) ;
#46909=DIRECTION ( 'NONE',  ( 0.000000000000000000, 1.846105847067148022E-16, -1.000000000000000000 ) ) ;
#46948=CARTESIAN_POINT ( 'NONE',  ( 184.1718750003414016, 9.264065473108010111E-16, -7.564683531250000925 ) ) ;
#47014=CARTESIAN_POINT ( 'NONE',  ( 184.2135416670080588, 4.367472073101518859, -7.564683531249999149 ) ) ;
#47049=ORIENTED_EDGE ( 'NONE', *, *, #62605, .T. ) ;
#47131=ADVANCED_FACE ( 'NONE', ( #37969 ), #49102, .T. ) ;
#47160=CARTESIAN_POINT ( 'NONE',  ( 187.5000000000000000, 1.500000000000000000, -6.000000000000000000 ) ) ;
#47188=CARTESIAN_POINT ( 'NONE',  ( 88.00000000000001421, 1.004210375300829477E-15, 8.199999999999999289 ) ) ;
#47191=CARTESIAN_POINT ( 'NONE',  ( 185.5729166673494603, 4.445597072760072876, -7.700000000000080114 ) ) ;
#47192=CIRCLE ( 'NONE', #101570, 3.000000000000000444 ) ;
#47257=VECTOR ( 'NONE', #58304, 1000.000000000000000 ) ;
#47296=CARTESIAN_POINT ( 'NONE',  ( 185.5000000000000000, 0.000000000000000000, 7.700000000000000178 ) ) ;
#47314=AXIS2_PLACEMENT_3D ( 'NONE', #99354, #1139, #61360 ) ;
#47418=CARTESIAN_POINT ( 'NONE',  ( 186.0000000000000000, 0.000000000000000000, 7.700000000000000178 ) ) ;
#47495=CARTESIAN_POINT ( 'NONE',  ( 184.7916666666666572, 4.445597072760062218, -7.700000000000102318 ) ) ;
#47539=CARTESIAN_POINT ( 'NONE',  ( 186.4010416670080588, -4.367472073101519747, 7.564683531249999149 ) ) ;
#47571=DIRECTION ( 'NONE',  ( 1.000000000000000000, 0.000000000000000000, 0.000000000000000000 ) ) ;
#47649=CARTESIAN_POINT ( 'NONE',  ( 187.5000000000000000, 0.000000000000000000, 7.700000000000000178 ) ) ;
#47654=CARTESIAN_POINT ( 'NONE',  ( 186.2135416670080588, 4.367472073101518859, -7.564683531249999149 ) ) ;
#47773=AXIS2_PLACEMENT_3D ( 'NONE', #18474, #109437, #117285 ) ;
#47840=CARTESIAN_POINT ( 'NONE',  ( 187.5000000000000000, 0.000000000000000000, 0.000000000000000000 ) ) ;
#47858=EDGE_CURVE ( 'NONE', #116188, #118850, #63256, .T. ) ;
#47882=SURFACE_STYLE_FILL_AREA ( #7931 ) ;
#47937=ORIENTED_EDGE ( 'NONE', *, *, #90954, .F. ) ;
#47941=CARTESIAN_POINT ( 'NONE',  ( 186.5000000000000000, 0.000000000000000000, 7.700000000000000178 ) ) ;
#48039=VECTOR ( 'NONE', #121272, 1000.000000000000000 ) ;
#48064=ORIENTED_EDGE ( 'NONE', *, *, #92781, .T. ) ;
#48065=CARTESIAN_POINT ( 'NONE',  ( 111.3047543057325584, 7.846687871447191931, -3.765660354317603709 ) ) ;
#48177=CARTESIAN_POINT ( 'NONE',  ( 184.0677083336747160, -4.367472073101514418, -7.564683531250002702 ) ) ;
#48244=CARTESIAN_POINT ( 'NONE',  ( 185.4583333333333428, 4.445597072760175905, 7.699999999999896261 ) ) ;
#48292=CARTESIAN_POINT ( 'NONE',  ( 185.2968750003414300, 8.734944146203032389, 5.348610694689227483E-16 ) ) ;
#48297=VERTEX_POINT ( 'NONE', #70996 ) ;
#48308=PLANE ( 'NONE',  #47314 ) ;
#48312=DIRECTION ( 'NONE',  ( -1.000000000000000000, -0.000000000000000000, -0.000000000000000000 ) ) ;
#48336=CARTESIAN_POINT ( 'NONE',  ( 111.9573209325854606, 7.065995906185201569, 3.073256371337414361 ) ) ;
#48366=VECTOR ( 'NONE', #94900, 1000.000000000000000 ) ;
#48375=CARTESIAN_POINT ( 'NONE',  ( 186.1510416670080588, 4.367472073101518859, -7.564683531249999149 ) ) ;
#48424=EDGE_CURVE ( 'NONE', #79874, #64073, #13984, .T. ) ;
#48445=CARTESIAN_POINT ( 'NONE',  ( 183.9218750003414016, 0.000000000000000000, 7.564683531250000925 ) ) ;
#48467=CARTESIAN_POINT ( 'NONE',  ( 187.5000000000000000, 0.000000000000000000, 8.699999999999999289 ) ) ;
#48514=CARTESIAN_POINT ( 'NONE',  ( 179.5000000000000000, -1.375000000000000000, 7.634788798650553154 ) ) ;
#48520=PLANE ( 'NONE',  #35142 ) ;
#48583=CARTESIAN_POINT ( 'NONE',  ( 184.5000000000000000, 0.000000000000000000, 7.700000000000000178 ) ) ;
#48616=CYLINDRICAL_SURFACE ( 'NONE', #83962, 7.700000000000000178 ) ;
#48628=CARTESIAN_POINT ( 'NONE',  ( 103.2649310519763617, 8.549820648965553715, -1.639149876075294276 ) ) ;
#48646=DIRECTION ( 'NONE',  ( -1.000000000000000000, -0.000000000000000000, -0.000000000000000000 ) ) ;
#48647=STYLED_ITEM ( 'NONE', ( #3452 ), #57499 ) ;
#48761=CARTESIAN_POINT ( 'NONE',  ( 127.5000000000000000, -1.500000000000000000, -6.000000000000000000 ) ) ;
#48772=CARTESIAN_POINT ( 'NONE',  ( 129.5000000000000000, -1.000000000000025535, -7.634788798650553154 ) ) ;
#48788=LINE ( 'NONE', #38994, #122376 ) ;
#48814=ADVANCED_FACE ( 'NONE', ( #91760 ), #102236, .T. ) ;
#48835=CARTESIAN_POINT ( 'NONE',  ( 184.6093750003413732, 9.264065473108010111E-16, -7.564683531250000925 ) ) ;
#48957=EDGE_LOOP ( 'NONE', ( #127374, #33632, #44144, #110091 ) ) ;
#49000=CARTESIAN_POINT ( 'NONE',  ( 110.5253642625963835, 6.372598327064348922, -4.327233595554000445 ) ) ;
#49030=EDGE_CURVE ( 'NONE', #94355, #44902, #97399, .T. ) ;
#49041=CARTESIAN_POINT ( 'NONE',  ( 185.6093750003413732, 9.264065473108010111E-16, -7.564683531250000925 ) ) ;
#49102=PLANE ( 'NONE',  #56456 ) ;
#49107=DIRECTION ( 'NONE',  ( 0.000000000000000000, -0.000000000000000000, 1.000000000000000000 ) ) ;
#49111=DIRECTION ( 'NONE',  ( 0.000000000000000000, 1.000000000000000000, 0.000000000000000000 ) ) ;
#49135=DIRECTION ( 'NONE',  ( -1.000000000000000000, -0.000000000000000000, -0.000000000000000000 ) ) ;
#49173=CARTESIAN_POINT ( 'NONE',  ( 107.6614812150378953, 5.855766388782979170, 4.999999999999952927 ) ) ;
#49181=CARTESIAN_POINT ( 'NONE',  ( 179.5000000000000000, 0.6250000000000000000, 7.634788798650556707 ) ) ;
#49194=ORIENTED_EDGE ( 'NONE', *, *, #31488, .F. ) ;
#49214=EDGE_LOOP ( 'NONE', ( #52904, #31692, #13433, #37798 ) ) ;
#49276=CARTESIAN_POINT ( 'NONE',  ( 183.9609375001707008, 0.000000000000000000, 7.632341765625000107 ) ) ;
#49290=CARTESIAN_POINT ( 'NONE',  ( 104.9451419649933115, 7.743416704392222627, -3.971277570916745603 ) ) ;
#49367=VERTEX_POINT ( 'NONE', #18034 ) ;
#49368=CARTESIAN_POINT ( 'NONE',  ( 112.9336158378006445, 8.661976086582759748, 0.8288528769330567592 ) ) ;
#49391=DIRECTION ( 'NONE',  ( -1.000000000000000000, -0.000000000000000000, -0.000000000000000000 ) ) ;
#49402=CARTESIAN_POINT ( 'NONE',  ( 184.4583333333333144, 4.445597072760201662, 7.699999999999855405 ) ) ;
#49487=CARTESIAN_POINT ( 'NONE',  ( 183.8593750003413732, 0.000000000000000000, 7.564683531250000925 ) ) ;
#49593=LINE ( 'NONE', #47649, #76128 ) ;
#49617=LINE ( 'NONE', #71823, #74006 ) ;
#49645=CARTESIAN_POINT ( 'NONE',  ( 108.3415395100210503, 5.863329682499133888, 4.991179557506976394 ) ) ;
#49675=LINE ( 'NONE', #58203, #117790 ) ;
#49694=VECTOR ( 'NONE', #5158, 1000.000000000000000 ) ;
#49709=CARTESIAN_POINT ( 'NONE',  ( 186.0729166673494603, 4.445597072760091528, -7.700000000000049916 ) ) ;
#49711=DIRECTION ( 'NONE',  ( 0.000000000000000000, -1.000000000000000000, -0.000000000000000000 ) ) ;
#49758=ORIENTED_EDGE ( 'NONE', *, *, #21592, .F. ) ;
#49803=DIRECTION ( 'NONE',  ( 1.000000000000000000, 0.000000000000000000, 0.000000000000000000 ) ) ;
#49911=CARTESIAN_POINT ( 'NONE',  ( 185.3229166673494888, -4.445597072760063107, 7.700000000000102318 ) ) ;
#49937=CARTESIAN_POINT ( 'NONE',  ( 106.3595851929959082, 7.300492252098111479, 4.734447472102021770 ) ) ;
#50012=CARTESIAN_POINT ( 'NONE',  ( 109.6376890251878251, 7.303981195022478445, 4.727079717527256086 ) ) ;
#50030=EDGE_CURVE ( 'NONE', #60931, #50358, #41421, .T. ) ;
#50047=CARTESIAN_POINT ( 'NONE',  ( 186.6302083336747160, -4.367472073101514418, -7.564683531250002702 ) ) ;
#50054=VECTOR ( 'NONE', #22685, 1000.000000000000000 ) ;
#50076=EDGE_CURVE ( 'NONE', #57186, #83312, #21108, .T. ) ;
#50117=VERTEX_POINT ( 'NONE', #120605 ) ;
#50128=CARTESIAN_POINT ( 'NONE',  ( 185.4843750003414300, -8.734944146203032389, -1.604583208406768146E-15 ) ) ;
#50146=CARTESIAN_POINT ( 'NONE',  ( 127.5000000000000000, -1.500000000000000000, -6.000000000000000000 ) ) ;
#50183=EDGE_CURVE ( 'NONE', #102067, #27968, #33527, .T. ) ;
#50186=VECTOR ( 'NONE', #4602, 1000.000000000000000 ) ;
#50202=( BOUNDED_CURVE ( )  B_SPLINE_CURVE ( 2, ( #60512, #49402, #51339, #101712, #19256, #921, #11381 ),
 .UNSPECIFIED., .F., .F. ) 
 B_SPLINE_CURVE_WITH_KNOTS ( ( 3, 2, 2, 3 ),
 ( 0.8571428571428578724, 0.8809523809523817084, 0.9047619047619054333, 0.9285714285714292693 ),
 .UNSPECIFIED. ) 
 CURVE ( )  GEOMETRIC_REPRESENTATION_ITEM ( )  RATIONAL_B_SPLINE_CURVE ( ( 0.9999999999999956701, 0.8660254037844430375, 1.000000000000000000, 0.8660254037844387076, 1.000000000000000000, 0.8660254037844349329, 1.000000000000003775 ) ) 
 REPRESENTATION_ITEM ( '' )  );
#50275=CARTESIAN_POINT ( 'NONE',  ( 109.3324905233811393, 5.996841997646892075, 4.830676265755256438 ) ) ;
#50287=CARTESIAN_POINT ( 'NONE',  ( 179.5000000000000000, 1.375000000000000000, 7.634788798650556707 ) ) ;
#50336=CARTESIAN_POINT ( 'NONE',  ( 186.1145833340161175, 6.668395609140177704, -3.849999999999998312 ) ) ;
#50358=VERTEX_POINT ( 'NONE', #55086 ) ;
#50394=CARTESIAN_POINT ( 'NONE',  ( 186.7395833340161175, 4.445597072760133273, 7.699999999999975309 ) ) ;
#50416=PLANE ( 'NONE',  #116267 ) ;
#50433=CARTESIAN_POINT ( 'NONE',  ( 107.3283321151400003, 5.885277908845356620, 4.965988341037961717 ) ) ;
#50480=ADVANCED_FACE ( 'NONE', ( #92614 ), #1008, .F. ) ;
#50542=CARTESIAN_POINT ( 'NONE',  ( 106.6791543986367259, 7.234036580820199624, 4.833745377036900770 ) ) ;
#50628=CARTESIAN_POINT ( 'NONE',  ( 112.8677677318791979, 8.624640698664421734, 1.154296164367282218 ) ) ;
#50629=VECTOR ( 'NONE', #5, 1000.000000000000000 ) ;
#50662=CARTESIAN_POINT ( 'NONE',  ( 186.0468750003414300, -8.734944146203032389, -1.604583208406768146E-15 ) ) ;
#50674=EDGE_CURVE ( 'NONE', #79091, #57186, #127292, .T. ) ;
#50722=CARTESIAN_POINT ( 'NONE',  ( 88.00000000000001421, 0.000000000000000000, 8.699999999999999289 ) ) ;
#50740=EDGE_LOOP ( 'NONE', ( #112354, #78034, #29935, #95284, #41915, #24794, #14228, #9087 ) ) ;
#50758=CARTESIAN_POINT ( 'NONE',  ( 185.4427083336747160, -6.551208109652278289, 3.782341765624995134 ) ) ;
#50942=FACE_OUTER_BOUND ( 'NONE', #48957, .T. ) ;
#50968=( BOUNDED_CURVE ( )  B_SPLINE_CURVE ( 2, ( #6801, #86682, #125955, #117402, #15994, #105021, #47418 ),
 .UNSPECIFIED., .F., .F. ) 
 B_SPLINE_CURVE_WITH_KNOTS ( ( 3, 2, 2, 3 ),
 ( 0.3571428571428574283, 0.3809523809523812643, 0.4047619047619051003, 0.4285714285714289362 ),
 .UNSPECIFIED. ) 
 CURVE ( )  GEOMETRIC_REPRESENTATION_ITEM ( )  RATIONAL_B_SPLINE_CURVE ( ( 0.9999999999999984457, 0.8660254037844402619, 1.000000000000000000, 0.8660254037844387076, 1.000000000000000000, 0.8660254037844364872, 1.000000000000002220 ) ) 
 REPRESENTATION_ITEM ( '' )  );
#50970=CARTESIAN_POINT ( 'NONE',  ( 187.1927083336747160, 6.551208109652275624, -3.782341765624998686 ) ) ;
#50991=CARTESIAN_POINT ( 'NONE',  ( 187.5000000000000000, 0.000000000000000000, 0.000000000000000000 ) ) ;
#51076=CARTESIAN_POINT ( 'NONE',  ( 184.7395833340161175, 4.445597072760175905, 7.699999999999896261 ) ) ;
#51195=VERTEX_POINT ( 'NONE', #39205 ) ;
#51215=CARTESIAN_POINT ( 'NONE',  ( 184.8177083336747160, 4.367472073101515306, 7.564683531250000925 ) ) ;
#51279=VERTEX_POINT ( 'NONE', #30665 ) ;
#51284=ORIENTED_EDGE ( 'NONE', *, *, #48424, .T. ) ;
#51332=CARTESIAN_POINT ( 'NONE',  ( 186.2552083336747444, 6.551208109652275624, -3.782341765624998686 ) ) ;
#51339=CARTESIAN_POINT ( 'NONE',  ( 184.4166666666666856, 6.668395609140176816, 3.850000000000000977 ) ) ;
#51564=CARTESIAN_POINT ( 'NONE',  ( 187.2395833340161460, 4.445597072760117285, 7.699999999999999289 ) ) ;
#51610=CARTESIAN_POINT ( 'NONE',  ( 184.7343750003414016, 8.734944146203032389, 5.348610694689227483E-16 ) ) ;
#51637=CARTESIAN_POINT ( 'NONE',  ( 127.5000000000000000, -1.500000000000000000, 6.000000000000000000 ) ) ;
#51645=FACE_OUTER_BOUND ( 'NONE', #90469, .T. ) ;
#51735=CARTESIAN_POINT ( 'NONE',  ( 103.0433693783451616, 7.671897681384138856, 0.6785423624469419934 ) ) ;
#51745=CARTESIAN_POINT ( 'NONE',  ( 179.5000000000000000, 0.000000000000000000, 6.000000000000000000 ) ) ;
#51756=EDGE_CURVE ( 'NONE', #21810, #3837, #69117, .T. ) ;
#51853=CARTESIAN_POINT ( 'NONE',  ( 184.9427083336747160, -6.551208109652278289, 3.782341765624995134 ) ) ;
#51882=CARTESIAN_POINT ( 'NONE',  ( 129.5000000000000000, 0.000000000000000000, 0.000000000000000000 ) ) ;
#52111=EDGE_LOOP ( 'NONE', ( #101636, #33699, #64668, #74661, #113552, #106522, #33375, #81195, #37257, #30188, #54161, #68466 ) ) ;
#52142=CARTESIAN_POINT ( 'NONE',  ( 186.5312500006828031, 9.429780353434619030E-16, -7.700000000000000178 ) ) ;
#52196=CARTESIAN_POINT ( 'NONE',  ( 186.7395833340161175, 4.445597072760117285, 7.699999999999999289 ) ) ;
#52204=VECTOR ( 'NONE', #17278, 1000.000000000000114 ) ;
#52248=CARTESIAN_POINT ( 'NONE',  ( 187.0468750003414300, -8.734944146203032389, -1.604583208406768146E-15 ) ) ;
#52421=CARTESIAN_POINT ( 'NONE',  ( 187.1979166673494603, 6.668395609140176816, 3.850000000000000977 ) ) ;
#52476=CARTESIAN_POINT ( 'NONE',  ( 185.5677083336747160, -4.367472073101514418, -7.564683531250002702 ) ) ;
#52503=CARTESIAN_POINT ( 'NONE',  ( 184.3645833340161175, -6.668395609140180369, 3.849999999999994760 ) ) ;
#52551=DIRECTION ( 'NONE',  ( 0.000000000000000000, 0.000000000000000000, -1.000000000000000000 ) ) ;
#52590=CARTESIAN_POINT ( 'NONE',  ( 187.2916666666666572, 4.445597072760120838, -7.699999999999998401 ) ) ;
#52606=AXIS2_PLACEMENT_3D ( 'NONE', #121464, #112951, #81560 ) ;
#52702=AXIS2_PLACEMENT_3D ( 'NONE', #72445, #35111, #64545 ) ;
#52840=CARTESIAN_POINT ( 'NONE',  ( 186.4062500006828031, -8.891194145520236347, -1.633285867636356693E-15 ) ) ;
#52852=PLANE ( 'NONE',  #15749 ) ;
#52865=VECTOR ( 'NONE', #120458, 1000.000000000000000 ) ;
#52889=CARTESIAN_POINT ( 'NONE',  ( 186.0885416670080872, -6.551208109652273848, -3.782341765625003571 ) ) ;
#52904=ORIENTED_EDGE ( 'NONE', *, *, #48424, .F. ) ;
#52961=DIRECTION ( 'NONE',  ( -1.000000000000000000, -0.000000000000000000, -0.000000000000000000 ) ) ;
#52962=CARTESIAN_POINT ( 'NONE',  ( 184.2500000000000000, 9.429780353434619030E-16, -7.700000000000000178 ) ) ;
#53137=CARTESIAN_POINT ( 'NONE',  ( 185.6093750003413732, 9.264065473108010111E-16, -7.564683531250000925 ) ) ;
#53217=CARTESIAN_POINT ( 'NONE',  ( 129.5000000000000000, -1.375000000000002442, -6.000000000000000888 ) ) ;
#53249=CARTESIAN_POINT ( 'NONE',  ( 184.1302083336747160, -4.367472073101514418, -7.564683531250002702 ) ) ;
#53268=AXIS2_PLACEMENT_3D ( 'NONE', #123529, #14215, #63980 ) ;
#53358=VECTOR ( 'NONE', #47571, 1000.000000000000000 ) ;
#53361=CARTESIAN_POINT ( 'NONE',  ( 179.5000000000000000, -0.6250000000000028866, -7.634788798650553154 ) ) ;
#53421=ORIENTED_EDGE ( 'NONE', *, *, #46588, .F. ) ;
#53433=CARTESIAN_POINT ( 'NONE',  ( 187.5000000000000000, 0.000000000000000000, 7.700000000000000178 ) ) ;
#53461=VECTOR ( 'NONE', #80066, 1000.000000000000000 ) ;
#53495=CARTESIAN_POINT ( 'NONE',  ( 187.1562500006828316, 8.891194145520236347, 5.444286225454521982E-16 ) ) ;
#53505=DIRECTION ( 'NONE',  ( 0.000000000000000000, -0.000000000000000000, -1.000000000000000000 ) ) ;
#53514=CIRCLE ( 'NONE', #57428, 0.5000000000000004441 ) ;
#53540=CARTESIAN_POINT ( 'NONE',  ( 186.4635416670080872, -4.367472073101519747, 7.564683531249999149 ) ) ;
#53607=CARTESIAN_POINT ( 'NONE',  ( 187.5000000000000000, 0.000000000000000000, 0.000000000000000000 ) ) ;
#53657=CARTESIAN_POINT ( 'NONE',  ( 108.0000000000000142, 5.855766388782936538, -5.000000000000004441 ) ) ;
#53727=ORIENTED_EDGE ( 'NONE', *, *, #70434, .F. ) ;
#53771=CARTESIAN_POINT ( 'NONE',  ( 184.4427083336747160, -6.551208109652278289, 3.782341765624995134 ) ) ;
#53773=CARTESIAN_POINT ( 'NONE',  ( 108.0000000000000142, 7.119691004531021328, -5.000000000000004441 ) ) ;
#53784=CARTESIAN_POINT ( 'NONE',  ( 87.50000000000001421, 0.000000000000000000, 7.700000000000000178 ) ) ;
#53790=CARTESIAN_POINT ( 'NONE',  ( 187.4609375001707008, 0.000000000000000000, 7.632341765625000107 ) ) ;
#53885=CARTESIAN_POINT ( 'NONE',  ( 184.7968750003414016, 8.734944146203032389, 5.348610694689227483E-16 ) ) ;
#54062=ORIENTED_EDGE ( 'NONE', *, *, #116007, .T. ) ;
#54101=LINE ( 'NONE', #91443, #80060 ) ;
#54130=CARTESIAN_POINT ( 'NONE',  ( 186.0312500006828031, 9.429780353434619030E-16, -7.700000000000000178 ) ) ;
#54141=DIRECTION ( 'NONE',  ( 0.000000000000000000, -1.000000000000000000, 0.000000000000000000 ) ) ;
#54161=ORIENTED_EDGE ( 'NONE', *, *, #40841, .F. ) ;
#54172=FACE_OUTER_BOUND ( 'NONE', #109540, .T. ) ;
#54182=CARTESIAN_POINT ( 'NONE',  ( 184.4635416670080588, -4.367472073101519747, 7.564683531249999149 ) ) ;
#54246=CARTESIAN_POINT ( 'NONE',  ( 187.0468750003414300, -8.734944146203032389, -1.604583208406767949E-15 ) ) ;
#54278=CARTESIAN_POINT ( 'NONE',  ( 186.8229166673494603, -4.445597072760107515, 7.700000000000023270 ) ) ;
#54408=EDGE_CURVE ( 'NONE', #64010, #43167, #19197, .T. ) ;
#54476=CARTESIAN_POINT ( 'NONE',  ( 179.5000000000000000, 1.375000000000002665, -7.634788798650556707 ) ) ;
#54485=VECTOR ( 'NONE', #19361, 1000.000000000000000 ) ;
#54512=CARTESIAN_POINT ( 'NONE',  ( 185.7968750003414300, 8.734944146203032389, 5.348610694689227483E-16 ) ) ;
#54535=CARTESIAN_POINT ( 'NONE',  ( 186.5000000000000000, 0.000000000000000000, 7.700000000000000178 ) ) ;
#54617=CARTESIAN_POINT ( 'NONE',  ( 184.5416666666666572, -4.445597072760039126, 7.700000000000142286 ) ) ;
#54660=AXIS2_PLACEMENT_3D ( 'NONE', #6158, #44826, #55282 ) ;
#54756=CARTESIAN_POINT ( 'NONE',  ( 185.0729166673494888, 4.445597072760120838, -7.699999999999998401 ) ) ;
#54803=CARTESIAN_POINT ( 'NONE',  ( 185.4635416670080872, -4.367472073101519747, 7.564683531249999149 ) ) ;
#54872=CARTESIAN_POINT ( 'NONE',  ( 186.4635416670080872, -4.367472073101520635, 7.564683531249999149 ) ) ;
#54922=CARTESIAN_POINT ( 'NONE',  ( 108.6749215142614275, 5.885800260617194191, -4.965357148327123937 ) ) ;
#54937=VECTOR ( 'NONE', #37247, 1000.000000000000000 ) ;
#55070=CARTESIAN_POINT ( 'NONE',  ( 187.5000000000000000, 0.000000000000000000, 7.700000000000000178 ) ) ;
#55086=CARTESIAN_POINT ( 'NONE',  ( 129.5000000000000000, -1.375000000000002665, -7.576237522675752345 ) ) ;
#55176=CARTESIAN_POINT ( 'NONE',  ( 185.1718750003414016, 9.264065473108010111E-16, -7.564683531250000925 ) ) ;
#55193=CARTESIAN_POINT ( 'NONE',  ( 87.50000000000001421, 1.034826545279513461E-15, 8.199999999999999289 ) ) ;
#55282=DIRECTION ( 'NONE',  ( 0.000000000000000000, 0.000000000000000000, 1.000000000000000000 ) ) ;
#55317=FACE_OUTER_BOUND ( 'NONE', #22873, .T. ) ;
#55350=LINE ( 'NONE', #95913, #83961 ) ;
#55391=CARTESIAN_POINT ( 'NONE',  ( 179.5000000000000000, 0.6250000000000000000, 7.634788798650556707 ) ) ;
#55407=VERTEX_POINT ( 'NONE', #74414 ) ;
#55422=CARTESIAN_POINT ( 'NONE',  ( 184.9062500006828031, -8.891194145520236347, -1.633285867636356693E-15 ) ) ;
#55466=CARTESIAN_POINT ( 'NONE',  ( 185.3385416670080872, 6.551208109652274736, 3.782341765625001351 ) ) ;
#55526=EDGE_CURVE ( 'NONE', #23165, #5682, #26602, .T. ) ;
#55601=DIRECTION ( 'NONE',  ( 0.000000000000000000, 1.000000000000000000, 0.000000000000000000 ) ) ;
#55639=VECTOR ( 'NONE', #56782, 1000.000000000000000 ) ;
#55710=EDGE_LOOP ( 'NONE', ( #95562, #64800, #38367, #24512 ) ) ;
#55765=ORIENTED_EDGE ( 'NONE', *, *, #20363, .T. ) ;
#55783=ADVANCED_FACE ( 'NONE', ( #36113 ), #15805, .T. ) ;
#55815=CARTESIAN_POINT ( 'NONE',  ( 184.2916666666666572, 4.445597072760120838, -7.699999999999998401 ) ) ;
#55951=AXIS2_PLACEMENT_3D ( 'NONE', #45951, #95049, #13887 ) ;
#55954=DIRECTION ( 'NONE',  ( 0.000000000000000000, 0.000000000000000000, 1.000000000000000000 ) ) ;
#55988=VECTOR ( 'NONE', #10812, 1000.000000000000000 ) ;
#56032=EDGE_LOOP ( 'NONE', ( #96080, #128165, #106419, #4989 ) ) ;
#56046=CARTESIAN_POINT ( 'NONE',  ( 184.1145833340161175, 6.668395609140177704, -3.849999999999998312 ) ) ;
#56094=CARTESIAN_POINT ( 'NONE',  ( 184.2135416670080588, 4.367472073101518859, -7.564683531249999149 ) ) ;
#56160=CARTESIAN_POINT ( 'NONE',  ( 185.0052083336747444, -6.551208109652278289, 3.782341765624995134 ) ) ;
#56290=VECTOR ( 'NONE', #18908, 1000.000000000000000 ) ;
#56382=ORIENTED_EDGE ( 'NONE', *, *, #85065, .T. ) ;
#56439=ORIENTED_EDGE ( 'NONE', *, *, #81594, .F. ) ;
#56449=CARTESIAN_POINT ( 'NONE',  ( 186.5833333333333144, -6.668395609140180369, 3.849999999999994760 ) ) ;
#56456=AXIS2_PLACEMENT_3D ( 'NONE', #68069, #66136, #107349 ) ;
#56481=CARTESIAN_POINT ( 'NONE',  ( 187.5000000000000000, 0.000000000000000000, 0.000000000000000000 ) ) ;
#56483=ADVANCED_FACE ( 'NONE', ( #92123 ), #81040, .T. ) ;
#56538=ORIENTED_EDGE ( 'NONE', *, *, #10269, .F. ) ;
#56638=CARTESIAN_POINT ( 'NONE',  ( 129.5000000000000000, -1.500000000000000000, -2.598076211353316900 ) ) ;
#56646=EDGE_CURVE ( 'NONE', #111056, #49367, #37142, .T. ) ;
#56647=ORIENTED_EDGE ( 'NONE', *, *, #91402, .F. ) ;
#56662=CARTESIAN_POINT ( 'NONE',  ( 186.7916666666667140, 4.445597072760099522, -7.700000000000035705 ) ) ;
#56680=CARTESIAN_POINT ( 'NONE',  ( 184.4895833340161460, -4.445597072760115509, -7.700000000000001954 ) ) ;
#56718=CARTESIAN_POINT ( 'NONE',  ( 184.9218750003414016, 0.000000000000000000, 7.564683531250000925 ) ) ;
#56740=DIRECTION ( 'NONE',  ( -1.000000000000000000, -0.000000000000000000, -0.000000000000000000 ) ) ;
#56782=DIRECTION ( 'NONE',  ( 0.000000000000000000, 0.000000000000000000, 1.000000000000000000 ) ) ;
#56790=CARTESIAN_POINT ( 'NONE',  ( 184.7968750003414584, 8.734944146203032389, 5.348610694689227483E-16 ) ) ;
#56849=EDGE_CURVE ( 'NONE', #64010, #100714, #97933, .T. ) ;
#56956=DIRECTION ( 'NONE',  ( 0.000000000000000000, 0.000000000000000000, -1.000000000000000000 ) ) ;
#57028=PRESENTATION_STYLE_ASSIGNMENT (( #77327 ) ) ;
#57062=CARTESIAN_POINT ( 'NONE',  ( 187.5000000000000000, 0.000000000000000000, 0.000000000000000000 ) ) ;
#57081=EDGE_CURVE ( 'NONE', #2046, #92765, #27599, .T. ) ;
#57101=CARTESIAN_POINT ( 'NONE',  ( 186.7083333333333428, -4.445597072760115509, -7.700000000000001954 ) ) ;
#57127=CARTESIAN_POINT ( 'NONE',  ( 185.3645833340161175, -6.668395609140180369, 3.849999999999994760 ) ) ;
#57155=CARTESIAN_POINT ( 'NONE',  ( 179.5000000000000000, -1.375000000000002442, -7.576237522675751457 ) ) ;
#57159=EDGE_LOOP ( 'NONE', ( #31790, #46166 ) ) ;
#57171=CARTESIAN_POINT ( 'NONE',  ( 127.5000000000000000, 0.000000000000000000, 0.000000000000000000 ) ) ;
#57186=VERTEX_POINT ( 'NONE', #57871 ) ;
#57295=CARTESIAN_POINT ( 'NONE',  ( 87.50000000000001421, 0.000000000000000000, 0.000000000000000000 ) ) ;
#57350=CARTESIAN_POINT ( 'NONE',  ( 186.4427083336747160, -6.551208109652278289, 3.782341765624995134 ) ) ;
#57424=ADVANCED_FACE ( 'NONE', ( #65586 ), #13251, .T. ) ;
#57428=AXIS2_PLACEMENT_3D ( 'NONE', #47188, #15103, #45896 ) ;
#57437=ORIENTED_EDGE ( 'NONE', *, *, #101185, .F. ) ;
#57459=ORIENTED_EDGE ( 'NONE', *, *, #95088, .F. ) ;
#57473=CARTESIAN_POINT ( 'NONE',  ( 183.9635416670080872, -4.367472073101520635, 7.564683531249999149 ) ) ;
#57498=PRODUCT ( 'Waterproof Outer Handle Shell', 'Waterproof Outer Handle Shell', '', ( #88257 ) ) ;
#57499=MANIFOLD_SOLID_BREP ( 'Cut-Extrude-Thin1', #79159 ) ;
#57508=VERTEX_POINT ( 'NONE', #95062 ) ;
#57521=CARTESIAN_POINT ( 'NONE',  ( 110.2425064135121744, 6.264065668498300710, -4.480648340451071299 ) ) ;
#57685=ORIENTED_EDGE ( 'NONE', *, *, #10603, .F. ) ;
#57763=CARTESIAN_POINT ( 'NONE',  ( 186.4583333333333144, 4.445597072760117285, 7.699999999999999289 ) ) ;
#57797=FACE_OUTER_BOUND ( 'NONE', #11758, .T. ) ;
#57806=CARTESIAN_POINT ( 'NONE',  ( 107.3288114731349197, 7.143999412540020799, -4.965851468055219264 ) ) ;
#57871=CARTESIAN_POINT ( 'NONE',  ( 187.5000000000000000, 1.065442715258197248E-15, -8.699999999999999289 ) ) ;
#57935=FACE_OUTER_BOUND ( 'NONE', #66862, .T. ) ;
#58000=ORIENTED_EDGE ( 'NONE', *, *, #15098, .T. ) ;
#58008=CARTESIAN_POINT ( 'NONE',  ( 185.4010416670080588, -4.367472073101519747, 7.564683531249999149 ) ) ;
#58122=CARTESIAN_POINT ( 'NONE',  ( 185.0468750003414300, -8.734944146203032389, -1.604583208406767949E-15 ) ) ;
#58203=CARTESIAN_POINT ( 'NONE',  ( 129.5000000000000000, -1.500000000000000000, 0.000000000000000000 ) ) ;
#58215=CARTESIAN_POINT ( 'NONE',  ( 186.6510416670080303, 4.367472073101518859, -7.564683531249999149 ) ) ;
#58276=FACE_OUTER_BOUND ( 'NONE', #4600, .T. ) ;
#58297=CARTESIAN_POINT ( 'NONE',  ( 179.5000000000000000, 0.000000000000000000, 0.000000000000000000 ) ) ;
#58304=DIRECTION ( 'NONE',  ( -1.000000000000000000, -0.000000000000000000, -0.000000000000000000 ) ) ;
#58413=CARTESIAN_POINT ( 'NONE',  ( 184.6666666666666856, -6.668395609140176816, -3.850000000000003642 ) ) ;
#58438=CARTESIAN_POINT ( 'NONE',  ( 185.5312500006828031, 9.429780353434619030E-16, -7.700000000000000178 ) ) ;
#58439=VECTOR ( 'NONE', #38856, 1000.000000000000000 ) ;
#58457=CARTESIAN_POINT ( 'NONE',  ( 186.6927083336747160, 6.551208109652275624, -3.782341765624998686 ) ) ;
#58537=CARTESIAN_POINT ( 'NONE',  ( 112.6717552496036205, 8.515422928616107612, 1.789336338813789506 ) ) ;
#58553=CARTESIAN_POINT ( 'NONE',  ( 184.2812500006828031, 0.000000000000000000, 7.700000000000000178 ) ) ;
#58650=CARTESIAN_POINT ( 'NONE',  ( 184.6510416670080588, 4.367472073101518859, -7.564683531249999149 ) ) ;
#58683=ORIENTED_EDGE ( 'NONE', *, *, #68426, .T. ) ;
#58758=CARTESIAN_POINT ( 'NONE',  ( 185.6302083336747444, -4.367472073101514418, -7.564683531250002702 ) ) ;
#58841=CARTESIAN_POINT ( 'NONE',  ( 185.7760416670080588, 6.551208109652274736, 3.782341765625001351 ) ) ;
#58862=EDGE_CURVE ( 'NONE', #12583, #64010, #103713, .T. ) ;
#58868=ORIENTED_EDGE ( 'NONE', *, *, #90237, .F. ) ;
#59096=CARTESIAN_POINT ( 'NONE',  ( 105.4748215620571301, 7.550127796438022010, 4.327541908659619629 ) ) ;
#59105=VERTEX_POINT ( 'NONE', #48772 ) ;
#59148=LINE ( 'NONE', #129197, #53461 ) ;
#59153=ORIENTED_EDGE ( 'NONE', *, *, #125392, .F. ) ;
#59179=CARTESIAN_POINT ( 'NONE',  ( 112.9994817707945032, 8.699702167353846605, -0.3436818946302461764 ) ) ;
#59191=ORIENTED_EDGE ( 'NONE', *, *, #21071, .T. ) ;
#59308=CARTESIAN_POINT ( 'NONE',  ( 184.1927083336747160, 6.551208109652275624, -3.782341765624998686 ) ) ;
#59427=CARTESIAN_POINT ( 'NONE',  ( 179.5000000000000000, 1.375000000000002442, -6.000000000000000888 ) ) ;
#59516=CARTESIAN_POINT ( 'NONE',  ( 185.5260416670080588, -6.551208109652273848, -3.782341765625003571 ) ) ;
#59542=ADVANCED_FACE ( 'NONE', ( #58276 ), #79831, .T. ) ;
#59545=LINE ( 'NONE', #9766, #42829 ) ;
#59603=ORIENTED_EDGE ( 'NONE', *, *, #90237, .T. ) ;
#59631=LINE ( 'NONE', #128369, #102860 ) ;
#59634=CARTESIAN_POINT ( 'NONE',  ( 88.00000000000001421, 0.000000000000000000, 0.000000000000000000 ) ) ;
#59646=CARTESIAN_POINT ( 'NONE',  ( 105.7578401975872282, 6.263922221111824840, 4.480854580342004567 ) ) ;
#59684=EDGE_CURVE ( 'NONE', #29124, #50358, #44420, .T. ) ;
#59757=CARTESIAN_POINT ( 'NONE',  ( 187.3593750003414016, 0.000000000000000000, 7.564683531250000925 ) ) ;
#59835=VERTEX_POINT ( 'NONE', #75174 ) ;
#59869=CARTESIAN_POINT ( 'NONE',  ( 187.2968750003414300, 8.734944146203032389, 5.348610694689227483E-16 ) ) ;
#59950=DIRECTION ( 'NONE',  ( 1.000000000000000000, 0.000000000000000000, 0.000000000000000000 ) ) ;
#59962=CARTESIAN_POINT ( 'NONE',  ( 185.6510416670080303, 4.367472073101518859, -7.564683531249999149 ) ) ;
#60112=CARTESIAN_POINT ( 'NONE',  ( 112.9920263949885566, 7.694814134679670126, 0.3288087409775817815 ) ) ;
#60153=CARTESIAN_POINT ( 'NONE',  ( 186.1093750003413732, 9.264065473108010111E-16, -7.564683531250000925 ) ) ;
#60205=ADVANCED_FACE ( 'NONE', ( #103839 ), #82271, .F. ) ;
#60214=DIRECTION ( 'NONE',  ( 0.000000000000000000, -1.000000000000000000, 0.000000000000000000 ) ) ;
#60229=DIRECTION ( 'NONE',  ( -0.4999999999999471534, -0.000000000000000000, 0.8660254037844692387 ) ) ;
#60243=CARTESIAN_POINT ( 'NONE',  ( 87.50000000000001421, 9.429780353434619030E-16, -7.700000000000000178 ) ) ;
#60247=EDGE_CURVE ( 'NONE', #66080, #128722, #81609, .T. ) ;
#60252=ORIENTED_EDGE ( 'NONE', *, *, #70570, .F. ) ;
#60398=CARTESIAN_POINT ( 'NONE',  ( 187.2760416670080588, 6.551208109652274736, 3.782341765625001351 ) ) ;
#60401=CARTESIAN_POINT ( 'NONE',  ( 107.6624854834585250, 7.119691004531023992, 5.000000000000003553 ) ) ;
#60477=CARTESIAN_POINT ( 'NONE',  ( 112.9654443591792159, 8.680014631837170924, -0.6741253490163554574 ) ) ;
#60503=CARTESIAN_POINT ( 'NONE',  ( 186.2135416670080872, 4.367472073101518859, -7.564683531249999149 ) ) ;
#60512=CARTESIAN_POINT ( 'NONE',  ( 184.5000000000000000, 0.000000000000000000, 7.700000000000000178 ) ) ;
#60596=CARTESIAN_POINT ( 'NONE',  ( 186.0677083336747444, -4.367472073101514418, -7.564683531250002702 ) ) ;
#60660=ORIENTED_EDGE ( 'NONE', *, *, #75964, .T. ) ;
#60682=DIRECTION ( 'NONE',  ( 0.000000000000000000, -1.000000000000000000, 0.000000000000000000 ) ) ;
#60765=CARTESIAN_POINT ( 'NONE',  ( 185.6249999999999716, -8.891194145520236347, -1.633285867636356299E-15 ) ) ;
#60778=CARTESIAN_POINT ( 'NONE',  ( 186.8177083336747160, 4.367472073101515306, 7.564683531250000925 ) ) ;
#60786=CARTESIAN_POINT ( 'NONE',  ( 183.8593750003413732, 0.000000000000000000, 7.564683531250000925 ) ) ;
#60871=EDGE_LOOP ( 'NONE', ( #129028, #3526, #9278, #100939 ) ) ;
#60931=VERTEX_POINT ( 'NONE', #57155 ) ;
#60958=EDGE_LOOP ( 'NONE', ( #102711, #42895, #47049, #126724 ) ) ;
#61009=CARTESIAN_POINT ( 'NONE',  ( 185.8177083336747160, 4.367472073101515306, 7.564683531250000925 ) ) ;
#61024=EDGE_LOOP ( 'NONE', ( #123188, #94821 ) ) ;
#61034=CARTESIAN_POINT ( 'NONE',  ( 187.5000000000000000, 1.065442715258197248E-15, -8.699999999999999289 ) ) ;
#61066=AXIS2_PLACEMENT_3D ( 'NONE', #3675, #71124, #41051 ) ;
#61097=EDGE_LOOP ( 'NONE', ( #80556, #8404, #117119, #89625, #56538 ) ) ;
#61128=CARTESIAN_POINT ( 'NONE',  ( 186.7135416670080872, 4.367472073101518859, -7.564683531249999149 ) ) ;
#61188=ORIENTED_EDGE ( 'NONE', *, *, #115199, .F. ) ;
#61359=DIRECTION ( 'NONE',  ( 0.000000000000000000, -1.000000000000000000, 0.000000000000000000 ) ) ;
#61360=DIRECTION ( 'NONE',  ( 0.000000000000000000, -0.000000000000000000, 1.000000000000000000 ) ) ;
#61437=CARTESIAN_POINT ( 'NONE',  ( 184.0260416670080588, -6.551208109652273848, -3.782341765625003571 ) ) ;
#61462=CARTESIAN_POINT ( 'NONE',  ( 186.1562500006828031, 8.891194145520236347, 5.444286225454521982E-16 ) ) ;
#61503=VECTOR ( 'NONE', #12118, 1000.000000000000000 ) ;
#61526=VECTOR ( 'NONE', #96236, 1000.000000000000000 ) ;
#61678=CARTESIAN_POINT ( 'NONE',  ( 185.8593750003413732, 0.000000000000000000, 7.564683531250000925 ) ) ;
#61688=AXIS2_PLACEMENT_3D ( 'NONE', #97408, #48312, #18196 ) ;
#61737=VERTEX_POINT ( 'NONE', #15458 ) ;
#61784=CARTESIAN_POINT ( 'NONE',  ( 179.5000000000000000, 0.000000000000000000, 0.000000000000000000 ) ) ;
#61789=CARTESIAN_POINT ( 'NONE',  ( 187.4218750003414016, 0.000000000000000000, 7.564683531250000925 ) ) ;
#61814=CARTESIAN_POINT ( 'NONE',  ( 107.9999999999992895, 5.855766388783293586, 5.000000000000080824 ) ) ;
#61824=CARTESIAN_POINT ( 'NONE',  ( 184.0312500006828031, 9.429780353434619030E-16, -7.700000000000000178 ) ) ;
#61873=EDGE_LOOP ( 'NONE', ( #61188, #56382, #101214, #73369 ) ) ;
#61898=CARTESIAN_POINT ( 'NONE',  ( 187.5000000000000000, 0.000000000000000000, 7.700000000000000178 ) ) ;
#61919=TOROIDAL_SURFACE ( 'NONE', #5448, 8.199999999999999289, 0.5000000000000000000 ) ;
#61949=CARTESIAN_POINT ( 'NONE',  ( 187.0000000000000000, 0.000000000000000000, 7.700000000000000178 ) ) ;
#62024=CARTESIAN_POINT ( 'NONE',  ( 185.8645833340161175, -6.668395609140180369, 3.849999999999994760 ) ) ;
#62074=CARTESIAN_POINT ( 'NONE',  ( 187.1718750003414016, 9.264065473108010111E-16, -7.564683531250000925 ) ) ;
#62222=LINE ( 'NONE', #32124, #127154 ) ;
#62239=ORIENTED_EDGE ( 'NONE', *, *, #110717, .T. ) ;
#62320=CARTESIAN_POINT ( 'NONE',  ( 184.2343750003414016, 8.734944146203032389, 5.348610694689227483E-16 ) ) ;
#62383=VERTEX_POINT ( 'NONE', #93099 ) ;
#62482=CARTESIAN_POINT ( 'NONE',  ( 179.5000000000000000, 1.375000000000000000, 7.576237522675751457 ) ) ;
#62520=PLANE ( 'NONE',  #77738 ) ;
#62524=CARTESIAN_POINT ( 'NONE',  ( 127.5000000000000000, 1.500000000000000000, 6.000000000000000000 ) ) ;
#62568=ORIENTED_EDGE ( 'NONE', *, *, #15719, .T. ) ;
#62605=EDGE_CURVE ( 'NONE', #83312, #73015, #128993, .T. ) ;
#62613=CARTESIAN_POINT ( 'NONE',  ( 108.0000000000000142, 8.700999999999998735, 0.000000000000000000 ) ) ;
#62717=EDGE_CURVE ( 'NONE', #77053, #5250, #110633, .T. ) ;
#62720=CARTESIAN_POINT ( 'NONE',  ( 184.9843750003414016, -8.734944146203032389, -1.604583208406768146E-15 ) ) ;
#62724=CARTESIAN_POINT ( 'NONE',  ( 179.5000000000000000, 0.6250000000000000000, 6.000000000000000000 ) ) ;
#62745=DIRECTION ( 'NONE',  ( 1.000000000000000000, 0.000000000000000000, 0.000000000000000000 ) ) ;
#62787=CARTESIAN_POINT ( 'NONE',  ( 187.0052083336747444, -6.551208109652278289, 3.782341765624995134 ) ) ;
#62830=LINE ( 'NONE', #63475, #52865 ) ;
#62897=EDGE_LOOP ( 'NONE', ( #24680, #60660, #118032, #68112 ) ) ;
#62947=CARTESIAN_POINT ( 'NONE',  ( 183.9010416670080588, -4.367472073101520635, 7.564683531249999149 ) ) ;
#62974=CARTESIAN_POINT ( 'NONE',  ( 184.5312500006828031, 9.429780353434619030E-16, -7.700000000000000178 ) ) ;
#63010=LINE ( 'NONE', #20521, #25466 ) ;
#63013=EDGE_CURVE ( 'NONE', #13525, #4435, #99559, .T. ) ;
#63016=ORIENTED_EDGE ( 'NONE', *, *, #118755, .T. ) ;
#63021=DIRECTION ( 'NONE',  ( 0.000000000000000000, 0.000000000000000000, -1.000000000000000000 ) ) ;
#63060=CARTESIAN_POINT ( 'NONE',  ( 185.1302083336747160, -4.367472073101514418, -7.564683531250002702 ) ) ;
#63162=EDGE_CURVE ( 'NONE', #129597, #94263, #3915, .T. ) ;
#63185=CARTESIAN_POINT ( 'NONE',  ( 127.5000000000000000, 9.429780353434619030E-16, -7.700000000000000178 ) ) ;
#63256=LINE ( 'NONE', #92063, #29201 ) ;
#63300=FACE_OUTER_BOUND ( 'NONE', #95338, .T. ) ;
#63330=EDGE_CURVE ( 'NONE', #16632, #68129, #65409, .T. ) ;
#63352=CARTESIAN_POINT ( 'NONE',  ( 186.1718750003414016, 9.264065473108010111E-16, -7.564683531250000925 ) ) ;
#63430=EDGE_CURVE ( 'NONE', #31133, #18092, #31783, .T. ) ;
#63447=CARTESIAN_POINT ( 'NONE',  ( 186.5729166673494888, 4.445597072760099522, -7.700000000000035705 ) ) ;
#63451=VECTOR ( 'NONE', #76366, 1000.000000000000000 ) ;
#63475=CARTESIAN_POINT ( 'NONE',  ( 187.5000000000000000, -1.500000000000000000, 6.000000000000000000 ) ) ;
#63478=ORIENTED_EDGE ( 'NONE', *, *, #24758, .F. ) ;
#63497=CARTESIAN_POINT ( 'NONE',  ( 129.5000000000000000, 9.429780353434619030E-16, -7.700000000000000178 ) ) ;
#63520=CARTESIAN_POINT ( 'NONE',  ( 185.9479166673494603, -6.668395609140176816, -3.850000000000003642 ) ) ;
#63567=( BOUNDED_CURVE ( )  B_SPLINE_CURVE ( 2, ( #82501, #73956, #32770, #13729, #112599, #72673, #22930 ),
 .UNSPECIFIED., .F., .F. ) 
 B_SPLINE_CURVE_WITH_KNOTS ( ( 3, 2, 2, 3 ),
 ( 0.6428571428571433488, 0.6666666666666670737, 0.6904761904761910207, 0.7142857142857148567 ),
 .UNSPECIFIED. ) 
 CURVE ( )  GEOMETRIC_REPRESENTATION_ITEM ( )  RATIONAL_B_SPLINE_CURVE ( ( 0.9999999999999974465, 0.8660254037844412611, 1.000000000000000000, 0.8660254037844387076, 1.000000000000000000, 0.8660254037844355990, 1.000000000000003109 ) ) 
 REPRESENTATION_ITEM ( '' )  );
#63604=CARTESIAN_POINT ( 'NONE',  ( 186.0260416670080588, -6.551208109652273848, -3.782341765625003571 ) ) ;
#63610=ADVANCED_FACE ( 'NONE', ( #65081 ), #103093, .T. ) ;
#63648=VERTEX_POINT ( 'NONE', #97787 ) ;
#63710=CARTESIAN_POINT ( 'NONE',  ( 184.8802083336747444, 4.367472073101515306, 7.564683531250000925 ) ) ;
#63724=VECTOR ( 'NONE', #16750, 1000.000000000000000 ) ;
#63745=ORIENTED_EDGE ( 'NONE', *, *, #13690, .T. ) ;
#63818=CARTESIAN_POINT ( 'NONE',  ( 184.5000000000000000, 0.000000000000000000, 7.700000000000000178 ) ) ;
#63820=UNCERTAINTY_MEASURE_WITH_UNIT (LENGTH_MEASURE( 1.000000000000000082E-05 ), #82675, 'distance_accuracy_value', 'NONE');
#63850=CARTESIAN_POINT ( 'NONE',  ( 184.2812500006828031, 0.000000000000000000, 7.700000000000000178 ) ) ;
#63852=CARTESIAN_POINT ( 'NONE',  ( 179.5000000000000000, 1.375000000000002665, -7.634788798650556707 ) ) ;
#63882=LINE ( 'NONE', #31852, #50054 ) ;
#63886=DIRECTION ( 'NONE',  ( 0.000000000000000000, 0.000000000000000000, -1.000000000000000000 ) ) ;
#63952=CARTESIAN_POINT ( 'NONE',  ( 185.7812500006828031, 0.000000000000000000, 7.700000000000000178 ) ) ;
#63980=DIRECTION ( 'NONE',  ( 0.000000000000000000, 0.000000000000000000, 1.000000000000000000 ) ) ;
#63994=CARTESIAN_POINT ( 'NONE',  ( 186.9218750003414016, 0.000000000000000000, 7.564683531250000925 ) ) ;
#64006=CARTESIAN_POINT ( 'NONE',  ( 186.3333333333333144, 6.668395609140177704, -3.849999999999998312 ) ) ;
#64010=VERTEX_POINT ( 'NONE', #23096 ) ;
#64062=CARTESIAN_POINT ( 'NONE',  ( 187.1718750003414016, 9.264065473108010111E-16, -7.564683531250000925 ) ) ;
#64073=VERTEX_POINT ( 'NONE', #17097 ) ;
#64152=ORIENTED_EDGE ( 'NONE', *, *, #50076, .F. ) ;
#64269=VECTOR ( 'NONE', #74122, 1000.000000000000000 ) ;
#64299=FILL_AREA_STYLE_COLOUR ( '', #40341 ) ;
#64329=( BOUNDED_CURVE ( )  B_SPLINE_CURVE ( 2, ( #44943, #15457, #94670, #124787, #35136, #56662, #95325 ),
 .UNSPECIFIED., .F., .F. ) 
 B_SPLINE_CURVE_WITH_KNOTS ( ( 3, 2, 2, 3 ),
 ( 0.1428571428571429880, 0.1666666666666668239, 0.1904761904761906322, 0.2142857142857144681 ),
 .UNSPECIFIED. ) 
 CURVE ( )  GEOMETRIC_REPRESENTATION_ITEM ( )  RATIONAL_B_SPLINE_CURVE ( ( 0.9999999999999992228, 0.8660254037844394848, 1.000000000000000000, 0.8660254037844387076, 1.000000000000000000, 0.8660254037844375974, 1.000000000000001110 ) ) 
 REPRESENTATION_ITEM ( '' )  );
#64345=CARTESIAN_POINT ( 'NONE',  ( 184.5052083336747444, -6.551208109652278289, 3.782341765624995134 ) ) ;
#64429=ORIENTED_EDGE ( 'NONE', *, *, #46588, .T. ) ;
#64515=ORIENTED_EDGE ( 'NONE', *, *, #35070, .F. ) ;
#64545=DIRECTION ( 'NONE',  ( 0.000000000000000000, 0.000000000000000000, 1.000000000000000000 ) ) ;
#64564=CARTESIAN_POINT ( 'NONE',  ( 187.5000000000000000, -1.500000000000000000, -6.000000000000000000 ) ) ;
#64585=CARTESIAN_POINT ( 'NONE',  ( 184.6979166673494603, 6.668395609140176816, 3.850000000000000977 ) ) ;
#64591=EDGE_CURVE ( 'NONE', #62383, #16557, #44506, .T. ) ;
#64632=CARTESIAN_POINT ( 'NONE',  ( 184.0468750003414300, -8.734944146203032389, -1.604583208406768146E-15 ) ) ;
#64668=ORIENTED_EDGE ( 'NONE', *, *, #110318, .F. ) ;
#64699=CARTESIAN_POINT ( 'NONE',  ( 186.6718750003414016, 9.264065473108010111E-16, -7.564683531250000925 ) ) ;
#64800=ORIENTED_EDGE ( 'NONE', *, *, #245, .T. ) ;
#64872=LINE ( 'NONE', #55070, #25481 ) ;
#64931=FILL_AREA_STYLE ('',( #64299 ) ) ;
#64975=CARTESIAN_POINT ( 'NONE',  ( 184.9218750003414016, 0.000000000000000000, 7.564683531250000925 ) ) ;
#64994=FACE_OUTER_BOUND ( 'NONE', #21079, .T. ) ;
#65026=DIRECTION ( 'NONE',  ( 0.000000000000000000, -1.000000000000000000, -0.000000000000000000 ) ) ;
#65058=ORIENTED_EDGE ( 'NONE', *, *, #57081, .F. ) ;
#65074=( BOUNDED_CURVE ( )  B_SPLINE_CURVE ( 2, ( #59757, #8039, #60398, #38160, #117995, #119942, #9985, #144, #40095, #29619, #28994, #28347, #108173, #99010, #18512, #129145, #58457, #9338, #39474, #30292, #79381, #100307, #98349, #119285, #4018, #70836, #100928, #21746, #72774, #21086, #1445, #43328, #63604, #43965, #33508, #110751, #61678, #61009, #83868, #11910, #12547, #121868, #53137, #52476, #93069, #73405, #11263, #92400, #113331, #30931, #2729, #23671, #32225, #72135, #41398, #42695, #82603, #112058, #51853, #103525, #13837, #51215, #2081, #111386, #91124, #101592, #91764, #22402, #81309, #3381, #53771, #121224, #42026, #93700, #31563, #62320, #83249, #122520, #123166, #71470, #81931, #102239, #32870, #62947, #112703 ),
 .UNSPECIFIED., .F., .F. ) 
 B_SPLINE_CURVE_WITH_KNOTS ( ( 3, 2, 2, 2, 2, 2, 2, 2, 2, 2, 2, 2, 2, 2, 2, 2, 2, 2, 2, 2, 2, 2, 2, 2, 2, 2, 2, 2, 2, 2, 2, 2, 2, 2, 2, 2, 2, 2, 2, 2, 2, 2, 3 ),
 ( 0.000000000000000000, 0.02380952380952380820, 0.04761904761904761640, 0.07142857142857142461, 0.09523809523809523281, 0.1190476190476190410, 0.1428571428571428492, 0.1666666666666666574, 0.1904761904761904656, 0.2142857142857142738, 0.2380952380952380820, 0.2619047619047619180, 0.2857142857142856984, 0.3095238095238095344, 0.3333333333333333148, 0.3571428571428571508, 0.3809523809523809312, 0.4047619047619047672, 0.4285714285714285476, 0.4523809523809523836, 0.4761904761904761640, 0.5000000000000000000, 0.5238095238095238360, 0.5476190476190476719, 0.5714285714285713969, 0.5952380952380952328, 0.6190476190476190688, 0.6428571428571429047, 0.6666666666666666297, 0.6904761904761904656, 0.7142857142857143016, 0.7380952380952381375, 0.7619047619047618625, 0.7857142857142856984, 0.8095238095238095344, 0.8333333333333333703, 0.8571428571428570953, 0.8809523809523809312, 0.9047619047619047672, 0.9285714285714286031, 0.9523809523809523281, 0.9761904761904761640, 1.000000000000000000 ),
 .UNSPECIFIED. ) 
 CURVE ( )  GEOMETRIC_REPRESENTATION_ITEM ( )  RATIONAL_B_SPLINE_CURVE ( ( 1.000000000000000000, 0.8660254037844387076, 1.000000000000000000, 0.8660254037844387076, 1.000000000000000000, 0.8660254037844387076, 1.000000000000000000, 0.8660254037844387076, 1.000000000000000000, 0.8660254037844387076, 1.000000000000000000, 0.8660254037844387076, 1.000000000000000000, 0.8660254037844387076, 1.000000000000000000, 0.8660254037844387076, 1.000000000000000000, 0.8660254037844387076, 1.000000000000000000, 0.8660254037844387076, 1.000000000000000000, 0.8660254037844387076, 1.000000000000000000, 0.8660254037844387076, 1.000000000000000000, 0.8660254037844387076, 1.000000000000000000, 0.8660254037844387076, 1.000000000000000000, 0.8660254037844387076, 1.000000000000000000, 0.8660254037844387076, 1.000000000000000000, 0.8660254037844387076, 1.000000000000000000, 0.8660254037844387076, 1.000000000000000000, 0.8660254037844387076, 1.000000000000000000, 0.8660254037844387076, 1.000000000000000000, 0.8660254037844387076, 1.000000000000000000, 0.8660254037844387076, 1.000000000000000000, 0.8660254037844387076, 1.000000000000000000, 0.8660254037844387076, 1.000000000000000000, 0.8660254037844387076, 1.000000000000000000, 0.8660254037844387076, 1.000000000000000000, 0.8660254037844387076, 1.000000000000000000, 0.8660254037844387076, 1.000000000000000000, 0.8660254037844387076, 1.000000000000000000, 0.8660254037844387076, 1.000000000000000000, 0.8660254037844387076, 1.000000000000000000, 0.8660254037844387076, 1.000000000000000000, 0.8660254037844387076, 1.000000000000000000, 0.8660254037844387076, 1.000000000000000000, 0.8660254037844387076, 1.000000000000000000, 0.8660254037844387076, 1.000000000000000000, 0.8660254037844387076, 1.000000000000000000, 0.8660254037844387076, 1.000000000000000000, 0.8660254037844387076, 1.000000000000000000, 0.8660254037844387076, 1.000000000000000000, 0.8660254037844387076, 1.000000000000000000, 0.8660254037844387076, 1.000000000000000000 ) ) 
 REPRESENTATION_ITEM ( '' )  );
#65081=FACE_OUTER_BOUND ( 'NONE', #62897, .T. ) ;
#65208=DIRECTION ( 'NONE',  ( 0.000000000000000000, -1.846105847067148515E-16, -1.000000000000000000 ) ) ;
#65219=CARTESIAN_POINT ( 'NONE',  ( 187.1927083336747160, 6.551208109652275624, -3.782341765624998686 ) ) ;
#65333=CARTESIAN_POINT ( 'NONE',  ( 187.3802083336747444, 4.367472073101515306, 7.564683531250000925 ) ) ;
#65341=ORIENTED_EDGE ( 'NONE', *, *, #22528, .T. ) ;
#65409=LINE ( 'NONE', #45792, #110448 ) ;
#65481=ORIENTED_EDGE ( 'NONE', *, *, #56849, .T. ) ;
#65586=FACE_OUTER_BOUND ( 'NONE', #61873, .T. ) ;
#65629=CARTESIAN_POINT ( 'NONE',  ( 187.3750000000000000, 8.891194145520236347, 5.444286225454521982E-16 ) ) ;
#65634=DIRECTION ( 'NONE',  ( -1.000000000000000000, -0.000000000000000000, -0.000000000000000000 ) ) ;
#65803=AXIS2_PLACEMENT_3D ( 'NONE', #1117, #71146, #31243 ) ;
#65876=CARTESIAN_POINT ( 'NONE',  ( 185.2812500006828031, 0.000000000000000000, 7.700000000000000178 ) ) ;
#65880=EDGE_LOOP ( 'NONE', ( #117429, #60252, #39720, #101765 ) ) ;
#65884=LINE ( 'NONE', #84884, #69706 ) ;
#65916=CARTESIAN_POINT ( 'NONE',  ( 185.5468750003414300, -8.734944146203032389, -1.604583208406768146E-15 ) ) ;
#65955=VERTEX_POINT ( 'NONE', #46453 ) ;
#65989=CARTESIAN_POINT ( 'NONE',  ( 185.4635416670080872, -4.367472073101520635, 7.564683531249999149 ) ) ;
#66040=CARTESIAN_POINT ( 'NONE',  ( 187.5000000000000000, 1.375000000000000000, 7.576237522675751457 ) ) ;
#66080=VERTEX_POINT ( 'NONE', #89613 ) ;
#66136=DIRECTION ( 'NONE',  ( 1.000000000000000000, 0.000000000000000000, 0.000000000000000000 ) ) ;
#66151=LINE ( 'NONE', #106088, #118320 ) ;
#66181=CARTESIAN_POINT ( 'NONE',  ( 187.5000000000000000, 0.000000000000000000, 0.000000000000000000 ) ) ;
#66228=LINE ( 'NONE', #113403, #35095 ) ;
#66233=ORIENTED_EDGE ( 'NONE', *, *, #97769, .T. ) ;
#66265=ADVANCED_FACE ( 'NONE', ( #121004, #72564 ), #112483, .F. ) ;
#66277=CARTESIAN_POINT ( 'NONE',  ( 184.6250000000000000, -8.891194145520236347, -1.633285867636356693E-15 ) ) ;
#66493=CARTESIAN_POINT ( 'NONE',  ( 185.5312500006828031, 9.429780353434619030E-16, -7.700000000000000178 ) ) ;
#66504=DIRECTION ( 'NONE',  ( 0.000000000000000000, -1.846105847067148515E-16, -1.000000000000000000 ) ) ;
#66511=CARTESIAN_POINT ( 'NONE',  ( 187.5000000000000000, 9.429780353434619030E-16, -7.700000000000000178 ) ) ;
#66513=CARTESIAN_POINT ( 'NONE',  ( 186.4843750003414016, -8.734944146203032389, -1.604583208406768146E-15 ) ) ;
#66527=LINE ( 'NONE', #116911, #101070 ) ;
#66543=CARTESIAN_POINT ( 'NONE',  ( 179.5000000000000000, -1.375000000000002442, -6.000000000000000888 ) ) ;
#66556=CARTESIAN_POINT ( 'NONE',  ( 184.7135416670080872, 4.367472073101518859, -7.564683531249999149 ) ) ;
#66610=DIRECTION ( 'NONE',  ( -1.000000000000000000, -0.000000000000000000, -0.000000000000000000 ) ) ;
#66622=LINE ( 'NONE', #106549, #55639 ) ;
#66628=CARTESIAN_POINT ( 'NONE',  ( 184.3802083336747444, 4.367472073101515306, 7.564683531250000925 ) ) ;
#66629=DIRECTION ( 'NONE',  ( -1.000000000000000000, -0.000000000000000000, -0.000000000000000000 ) ) ;
#66689=CARTESIAN_POINT ( 'NONE',  ( 179.5000000000000000, 0.6250000000000000000, 7.634788798650556707 ) ) ;
#66700=CARTESIAN_POINT ( 'NONE',  ( 187.0833333333333144, -6.668395609140180369, 3.849999999999994760 ) ) ;
#66759=FACE_OUTER_BOUND ( 'NONE', #6176, .T. ) ;
#66836=CARTESIAN_POINT ( 'NONE',  ( 179.5000000000000000, -0.6250000000000000000, 7.634788798650553154 ) ) ;
#66862=EDGE_LOOP ( 'NONE', ( #125372, #114108, #39441, #119555 ) ) ;
#66909=CARTESIAN_POINT ( 'NONE',  ( 184.3750000000000000, 8.891194145520236347, 5.444286225454521982E-16 ) ) ;
#66961=ORIENTED_EDGE ( 'NONE', *, *, #15098, .F. ) ;
#67138=CARTESIAN_POINT ( 'NONE',  ( 183.8229166673494888, -4.445597072760122614, 7.699999999999998401 ) ) ;
#67177=CARTESIAN_POINT ( 'NONE',  ( 185.4218750003414016, 0.000000000000000000, 7.564683531250000925 ) ) ;
#67202=ORIENTED_EDGE ( 'NONE', *, *, #24597, .T. ) ;
#67243=CARTESIAN_POINT ( 'NONE',  ( 184.6302083336747444, -4.367472073101514418, -7.564683531250002702 ) ) ;
#67257=DIRECTION ( 'NONE',  ( 0.000000000000000000, 1.846105847067148022E-16, -1.000000000000000000 ) ) ;
#67273=VECTOR ( 'NONE', #83514, 1000.000000000000000 ) ;
#67372=CARTESIAN_POINT ( 'NONE',  ( 129.5000000000000000, 0.000000000000000000, 0.000000000000000000 ) ) ;
#67375=DIRECTION ( 'NONE',  ( -1.000000000000000000, -0.000000000000000000, -0.000000000000000000 ) ) ;
#67409=PLANE ( 'NONE',  #89234 ) ;
#67429=LINE ( 'NONE', #37378, #50629 ) ;
#67492=ORIENTED_EDGE ( 'NONE', *, *, #88137, .T. ) ;
#67535=ORIENTED_EDGE ( 'NONE', *, *, #95088, .T. ) ;
#67549=CARTESIAN_POINT ( 'NONE',  ( 185.8333333333333144, 6.668395609140177704, -3.849999999999998312 ) ) ;
#67681=CARTESIAN_POINT ( 'NONE',  ( 110.2384023472883143, 7.457657641414515481, -4.482797374978448879 ) ) ;
#67688=ORIENTED_EDGE ( 'NONE', *, *, #50674, .F. ) ;
#67712=DIRECTION ( 'NONE',  ( 1.000000000000000000, 0.000000000000000000, 0.000000000000000000 ) ) ;
#67734=DIRECTION ( 'NONE',  ( 0.000000000000000000, -0.000000000000000000, -1.000000000000000000 ) ) ;
#67809=CARTESIAN_POINT ( 'NONE',  ( 186.1927083336747160, 6.551208109652275624, -3.782341765624998686 ) ) ;
#67923=CARTESIAN_POINT ( 'NONE',  ( 184.1718750003414016, 9.264065473108010111E-16, -7.564683531250000925 ) ) ;
#67944=LINE ( 'NONE', #127522, #97181 ) ;
#67964=CARTESIAN_POINT ( 'NONE',  ( 112.7330628718930967, 7.528728208595681259, 1.645054351054255237 ) ) ;
#68008=CARTESIAN_POINT ( 'NONE',  ( 187.0677083336747444, -4.367472073101514418, -7.564683531250002702 ) ) ;
#68060=CARTESIAN_POINT ( 'NONE',  ( 179.5000000000000000, -1.375000000000000000, 7.576237522675751457 ) ) ;
#68069=CARTESIAN_POINT ( 'NONE',  ( 129.5000000000000000, 0.000000000000000000, 0.000000000000000000 ) ) ;
#68076=DIRECTION ( 'NONE',  ( 1.000000000000000000, 0.000000000000000000, -0.000000000000000000 ) ) ;
#68112=ORIENTED_EDGE ( 'NONE', *, *, #68730, .F. ) ;
#68116=DIRECTION ( 'NONE',  ( 0.000000000000000000, 1.000000000000000000, -1.846105847067148761E-16 ) ) ;
#68129=VERTEX_POINT ( 'NONE', #10845 ) ;
#68184=DIRECTION ( 'NONE',  ( -1.000000000000000000, -0.000000000000000000, -0.000000000000000000 ) ) ;
#68204=CARTESIAN_POINT ( 'NONE',  ( 184.7500000000000000, 9.429780353434619030E-16, -7.700000000000000178 ) ) ;
#68253=CARTESIAN_POINT ( 'NONE',  ( 108.0000000000000142, 7.119691004531020440, 5.000000000000004441 ) ) ;
#68281=CIRCLE ( 'NONE', #107995, 3.000000000000000444 ) ;
#68426=EDGE_CURVE ( 'NONE', #61737, #128722, #47192, .T. ) ;
#68447=CARTESIAN_POINT ( 'NONE',  ( 185.6093750003413732, 9.264065473108010111E-16, -7.564683531250000925 ) ) ;
#68466=ORIENTED_EDGE ( 'NONE', *, *, #96973, .F. ) ;
#68486=DIRECTION ( 'NONE',  ( 1.000000000000000000, 0.000000000000000000, 0.000000000000000000 ) ) ;
#68560=DIRECTION ( 'NONE',  ( -1.000000000000000000, -0.000000000000000000, -0.000000000000000000 ) ) ;
#68564=CARTESIAN_POINT ( 'NONE',  ( 185.2552083336747444, 6.551208109652275624, -3.782341765624998686 ) ) ;
#68582=ORIENTED_EDGE ( 'NONE', *, *, #47858, .T. ) ;
#68593=ORIENTED_EDGE ( 'NONE', *, *, #82357, .T. ) ;
#68611=CARTESIAN_POINT ( 'NONE',  ( 111.7537803698471777, 6.952973673849077940, 3.318088645774402323 ) ) ;
#68617=EDGE_CURVE ( 'NONE', #26322, #8359, #32725, .T. ) ;
#68656=FACE_OUTER_BOUND ( 'NONE', #8955, .T. ) ;
#68703=AXIS2_PLACEMENT_3D ( 'NONE', #2922, #122685, #83418 ) ;
#68730=EDGE_CURVE ( 'NONE', #7606, #64073, #107480, .T. ) ;
#68746=ORIENTED_EDGE ( 'NONE', *, *, #74034, .T. ) ;
#68799=CARTESIAN_POINT ( 'NONE',  ( 185.8333333333333144, 6.668395609140177704, -3.849999999999998312 ) ) ;
#68854=CARTESIAN_POINT ( 'NONE',  ( 185.7083333333333428, -4.445597072760115509, -7.700000000000001954 ) ) ;
#68888=DIRECTION ( 'NONE',  ( -1.000000000000000000, -0.000000000000000000, -0.000000000000000000 ) ) ;
#68900=CARTESIAN_POINT ( 'NONE',  ( 104.2422576842260895, 8.047964328330300177, 3.313773385403227412 ) ) ;
#68944=CARTESIAN_POINT ( 'NONE',  ( 185.2500000000000000, 9.429780353434619030E-16, -7.700000000000000178 ) ) ;
#69094=CARTESIAN_POINT ( 'NONE',  ( 184.5677083336747444, -4.367472073101514418, -7.564683531250002702 ) ) ;
#69117=LINE ( 'NONE', #109027, #54485 ) ;
#69132=VERTEX_POINT ( 'NONE', #22968 ) ;
#69212=ORIENTED_EDGE ( 'NONE', *, *, #113984, .T. ) ;
#69283=CARTESIAN_POINT ( 'NONE',  ( 186.8593750003414016, 0.000000000000000000, 7.564683531250000925 ) ) ;
#69290=CARTESIAN_POINT ( 'NONE',  ( 129.5000000000000000, -1.500000000000000000, 0.000000000000000000 ) ) ;
#69318=ORIENTED_EDGE ( 'NONE', *, *, #97705, .F. ) ;
#69379=CIRCLE ( 'NONE', #115331, 7.700000000000000178 ) ;
#69419=CARTESIAN_POINT ( 'NONE',  ( 106.2064113537864927, 6.122648159495343911, 4.670050787261943448 ) ) ;
#69430=( NAMED_UNIT ( * ) SI_UNIT ( $, .STERADIAN. ) SOLID_ANGLE_UNIT ( ) );
#69435=DIRECTION ( 'NONE',  ( -0.000000000000000000, 1.000000000000000000, 1.846105847067148022E-16 ) ) ;
#69479=VERTEX_POINT ( 'NONE', #124062 ) ;
#69495=CYLINDRICAL_SURFACE ( 'NONE', #47773, 7.700000000000000178 ) ;
#69614=FACE_OUTER_BOUND ( 'NONE', #25043, .T. ) ;
#69624=CARTESIAN_POINT ( 'NONE',  ( 113.0002503959617144, 8.700143905611811945, 0.1604050591010280913 ) ) ;
#69706=VECTOR ( 'NONE', #124821, 1000.000000000000000 ) ;
#69747=CARTESIAN_POINT ( 'NONE',  ( 185.9427083336747160, -6.551208109652278289, 3.782341765624995134 ) ) ;
#69832=ADVANCED_FACE ( 'NONE', ( #40872 ), #37586, .F. ) ;
#69914=CARTESIAN_POINT ( 'NONE',  ( 111.9564666233451504, 7.065552756683692870, -3.073909748344711979 ) ) ;
#69955=CARTESIAN_POINT ( 'NONE',  ( 185.1927083336747160, 6.551208109652275624, -3.782341765624998686 ) ) ;
#69991=VECTOR ( 'NONE', #23910, 1000.000000000000000 ) ;
#70064=FACE_OUTER_BOUND ( 'NONE', #60871, .T. ) ;
#70192=ORIENTED_EDGE ( 'NONE', *, *, #45844, .T. ) ;
#70353=LINE ( 'NONE', #91929, #17398 ) ;
#70362=ORIENTED_EDGE ( 'NONE', *, *, #50183, .T. ) ;
#70392=VECTOR ( 'NONE', #82291, 1000.000000000000000 ) ;
#70396=CARTESIAN_POINT ( 'NONE',  ( 185.0260416670080588, -6.551208109652273848, -3.782341765625003571 ) ) ;
#70434=EDGE_CURVE ( 'NONE', #94355, #86071, #123595, .T. ) ;
#70570=EDGE_CURVE ( 'NONE', #1000, #109625, #118639, .T. ) ;
#70595=CARTESIAN_POINT ( 'NONE',  ( 185.1093750003413732, 9.264065473108010111E-16, -7.564683531250000925 ) ) ;
#70641=ORIENTED_EDGE ( 'NONE', *, *, #14397, .T. ) ;
#70655=AXIS2_PLACEMENT_3D ( 'NONE', #104286, #25715, #104905 ) ;
#70696=CARTESIAN_POINT ( 'NONE',  ( 184.6562500006828031, 8.891194145520236347, 5.444286225454521982E-16 ) ) ;
#70720=CARTESIAN_POINT ( 'NONE',  ( 106.8360844680885862, 5.968126920954556880, 4.865526191718072546 ) ) ;
#70760=DIRECTION ( 'NONE',  ( -1.000000000000000000, -0.000000000000000000, -0.000000000000000000 ) ) ;
#70789=CARTESIAN_POINT ( 'NONE',  ( 184.0833333333333144, -6.668395609140180369, 3.849999999999994760 ) ) ;
#70818=ORIENTED_EDGE ( 'NONE', *, *, #96973, .T. ) ;
#70836=CARTESIAN_POINT ( 'NONE',  ( 186.3177083336747160, 4.367472073101515306, 7.564683531250000925 ) ) ;
#70869=CARTESIAN_POINT ( 'NONE',  ( 184.4479166673494603, -6.668395609140176816, -3.850000000000003642 ) ) ;
#70921=CARTESIAN_POINT ( 'NONE',  ( 108.0000000000000142, 7.119691004531020440, 5.000000000000004441 ) ) ;
#70947=CARTESIAN_POINT ( 'NONE',  ( 185.9635416670080872, -4.367472073101519747, 7.564683531249999149 ) ) ;
#70996=CARTESIAN_POINT ( 'NONE',  ( 108.0000000000000142, 7.119691004531020440, 5.000000000000004441 ) ) ;
#71006=ADVANCED_FACE ( 'NONE', ( #69614 ), #11818, .F. ) ;
#71078=ORIENTED_EDGE ( 'NONE', *, *, #99521, .T. ) ;
#71095=ORIENTED_EDGE ( 'NONE', *, *, #43347, .T. ) ;
#71124=DIRECTION ( 'NONE',  ( 0.000000000000000000, 0.000000000000000000, 1.000000000000000000 ) ) ;
#71146=DIRECTION ( 'NONE',  ( -1.000000000000000000, -0.000000000000000000, -0.000000000000000000 ) ) ;
#71157=CARTESIAN_POINT ( 'NONE',  ( 129.5000000000000000, -1.500000000000000000, 2.598076211353316900 ) ) ;
#71182=CARTESIAN_POINT ( 'NONE',  ( 179.5000000000000000, -1.375000000000000222, 6.000000000000000000 ) ) ;
#71228=CARTESIAN_POINT ( 'NONE',  ( 186.5052083336747444, -6.551208109652278289, 3.782341765624995134 ) ) ;
#71390=CARTESIAN_POINT ( 'NONE',  ( 187.5000000000000000, 0.000000000000000000, 0.000000000000000000 ) ) ;
#71463=ORIENTED_EDGE ( 'NONE', *, *, #125351, .F. ) ;
#71470=CARTESIAN_POINT ( 'NONE',  ( 184.0677083336747160, -4.367472073101514418, -7.564683531250002702 ) ) ;
#71583=LINE ( 'NONE', #99125, #22891 ) ;
#71590=CARTESIAN_POINT ( 'NONE',  ( 187.0052083336747444, -6.551208109652278289, 3.782341765624995134 ) ) ;
#71695=EDGE_CURVE ( 'NONE', #80059, #69479, #122064, .T. ) ;
#71728=EDGE_LOOP ( 'NONE', ( #100071, #6152, #15492, #93256 ) ) ;
#71823=CARTESIAN_POINT ( 'NONE',  ( 129.5000000000000000, 1.375000000000002665, -7.634788798650556707 ) ) ;
#71845=CARTESIAN_POINT ( 'NONE',  ( 187.0312500006828031, 9.429780353434619030E-16, -7.700000000000000178 ) ) ;
#71895=CARTESIAN_POINT ( 'NONE',  ( 184.3177083336747160, 4.367472073101515306, 7.564683531250000925 ) ) ;
#72024=CARTESIAN_POINT ( 'NONE',  ( 103.1711462153774903, 7.589803906595561145, 1.339608020536842581 ) ) ;
#72071=DIRECTION ( 'NONE',  ( 0.000000000000000000, 0.000000000000000000, 1.000000000000000000 ) ) ;
#72127=PLANE ( 'NONE',  #8285 ) ;
#72135=CARTESIAN_POINT ( 'NONE',  ( 185.1510416670080872, 4.367472073101518859, -7.564683531249999149 ) ) ;
#72146=ADVANCED_FACE ( 'NONE', ( #2074 ), #72127, .T. ) ;
#72185=AXIS2_PLACEMENT_3D ( 'NONE', #66181, #104805, #76006 ) ;
#72249=DIRECTION ( 'NONE',  ( -1.000000000000000000, 0.000000000000000000, 0.000000000000000000 ) ) ;
#72288=CARTESIAN_POINT ( 'NONE',  ( 183.8229166673494319, -4.445597072760122614, 7.699999999999997513 ) ) ;
#72351=CARTESIAN_POINT ( 'NONE',  ( 187.5000000000000000, 0.000000000000000000, 7.700000000000000178 ) ) ;
#72445=CARTESIAN_POINT ( 'NONE',  ( 179.5000000000000000, 0.000000000000000000, 0.000000000000000000 ) ) ;
#72493=CARTESIAN_POINT ( 'NONE',  ( 186.4895833340161175, -4.445597072760115509, -7.700000000000001954 ) ) ;
#72496=EDGE_CURVE ( 'NONE', #33663, #63648, #100607, .T. ) ;
#72539=CARTESIAN_POINT ( 'NONE',  ( 186.6302083336747160, -4.367472073101514418, -7.564683531250002702 ) ) ;
#72545=AXIS2_PLACEMENT_3D ( 'NONE', #59634, #49803, #32 ) ;
#72564=FACE_BOUND ( 'NONE', #20887, .T. ) ;
#72603=CARTESIAN_POINT ( 'NONE',  ( 186.9218750003414016, 0.000000000000000000, 7.564683531250000925 ) ) ;
#72610=LINE ( 'NONE', #81142, #37104 ) ;
#72625=EDGE_CURVE ( 'NONE', #69132, #18092, #41084, .T. ) ;
#72631=EDGE_LOOP ( 'NONE', ( #2265, #112330, #76661, #30189 ) ) ;
#72649=EDGE_LOOP ( 'NONE', ( #17988, #1098, #12733, #128855 ) ) ;
#72656=DIRECTION ( 'NONE',  ( -1.000000000000000000, -0.000000000000000000, -0.000000000000000000 ) ) ;
#72673=CARTESIAN_POINT ( 'NONE',  ( 184.8229166673494888, -4.445597072760063107, 7.700000000000102318 ) ) ;
#72726=ADVANCED_FACE ( 'NONE', ( #15442 ), #76322, .F. ) ;
#72770=DIRECTION ( 'NONE',  ( 1.000000000000000000, 0.000000000000000000, 0.000000000000000000 ) ) ;
#72774=CARTESIAN_POINT ( 'NONE',  ( 186.1927083336747160, 6.551208109652275624, -3.782341765624998686 ) ) ;
#72884=CARTESIAN_POINT ( 'NONE',  ( 185.0468750003414016, -8.734944146203032389, -1.604583208406768146E-15 ) ) ;
#72993=DIRECTION ( 'NONE',  ( -1.000000000000000000, 0.000000000000000000, -0.000000000000000000 ) ) ;
#73015=VERTEX_POINT ( 'NONE', #50722 ) ;
#73033=CARTESIAN_POINT ( 'NONE',  ( 129.5000000000000000, 0.9999999999999985567, -7.634788798650556707 ) ) ;
#73038=AXIS2_PLACEMENT_3D ( 'NONE', #25332, #113077, #123536 ) ;
#73081=PLANE ( 'NONE',  #52702 ) ;
#73085=DIRECTION ( 'NONE',  ( 1.000000000000000000, 0.000000000000000000, 0.000000000000000000 ) ) ;
#73090=VECTOR ( 'NONE', #56740, 1000.000000000000000 ) ;
#73097=DIRECTION ( 'NONE',  ( 0.000000000000000000, 1.846105847067148022E-16, -1.000000000000000000 ) ) ;
#73107=EDGE_CURVE ( 'NONE', #29124, #1392, #3554, .T. ) ;
#73173=CARTESIAN_POINT ( 'NONE',  ( 186.7135416670080872, 4.367472073101518859, -7.564683531249999149 ) ) ;
#73260=CARTESIAN_POINT ( 'NONE',  ( 186.7812500006828031, 0.000000000000000000, 7.700000000000000178 ) ) ;
#73289=CARTESIAN_POINT ( 'NONE',  ( 103.0080513606563244, 7.694763653578461593, -0.3299518301331845205 ) ) ;
#73316=PRODUCT_DEFINITION_SHAPE ( 'NONE', 'NONE',  #88428 ) ;
#73328=ORIENTED_EDGE ( 'NONE', *, *, #63162, .F. ) ;
#73369=ORIENTED_EDGE ( 'NONE', *, *, #1629, .T. ) ;
#73405=CARTESIAN_POINT ( 'NONE',  ( 185.4843750003414016, -8.734944146203032389, -1.604583208406767949E-15 ) ) ;
#73438=ORIENTED_EDGE ( 'NONE', *, *, #111619, .F. ) ;
#73512=CARTESIAN_POINT ( 'NONE',  ( 185.2552083336747444, 6.551208109652275624, -3.782341765624998686 ) ) ;
#73548=ORIENTED_EDGE ( 'NONE', *, *, #123557, .F. ) ;
#73604=CARTESIAN_POINT ( 'NONE',  ( 187.5000000000000000, 0.000000000000000000, 0.000000000000000000 ) ) ;
#73643=EDGE_LOOP ( 'NONE', ( #117359, #114388, #33668, #28202 ) ) ;
#73727=DIRECTION ( 'NONE',  ( 0.000000000000000000, 1.000000000000000000, 0.000000000000000000 ) ) ;
#73731=EDGE_LOOP ( 'NONE', ( #97228, #70192, #58000, #99390 ) ) ;
#73751=CARTESIAN_POINT ( 'NONE',  ( 186.1562500006828031, 8.891194145520236347, 5.444286225454521982E-16 ) ) ;
#73776=DIRECTION ( 'NONE',  ( 0.000000000000000000, 0.000000000000000000, -1.000000000000000000 ) ) ;
#73803=CARTESIAN_POINT ( 'NONE',  ( 183.9427083336747160, -6.551208109652278289, 3.782341765624995134 ) ) ;
#73956=CARTESIAN_POINT ( 'NONE',  ( 184.9895833340161175, -4.445597072760163471, -7.699999999999919353 ) ) ;
#74006=VECTOR ( 'NONE', #61359, 1000.000000000000000 ) ;
#74034=EDGE_CURVE ( 'NONE', #116188, #59835, #122823, .T. ) ;
#74044=DIRECTION ( 'NONE',  ( 0.000000000000000000, 1.846105847067148022E-16, -1.000000000000000000 ) ) ;
#74122=DIRECTION ( 'NONE',  ( -1.000000000000000000, -0.000000000000000000, -0.000000000000000000 ) ) ;
#74170=FACE_OUTER_BOUND ( 'NONE', #26701, .T. ) ;
#74171=DIRECTION ( 'NONE',  ( 1.000000000000000000, 0.000000000000000000, 0.000000000000000000 ) ) ;
#74172=CARTESIAN_POINT ( 'NONE',  ( 185.0885416670080872, -6.551208109652273848, -3.782341765625003571 ) ) ;
#74252=ORIENTED_EDGE ( 'NONE', *, *, #99174, .F. ) ;
#74282=ORIENTED_EDGE ( 'NONE', *, *, #63013, .F. ) ;
#74365=VERTEX_POINT ( 'NONE', #89535 ) ;
#74414=CARTESIAN_POINT ( 'NONE',  ( 127.5000000000000000, 0.000000000000000000, 7.700000000000000178 ) ) ;
#74418=CARTESIAN_POINT ( 'NONE',  ( 186.8645833340161175, -6.668395609140180369, 3.849999999999994760 ) ) ;
#74461=CARTESIAN_POINT ( 'NONE',  ( 184.8802083336747444, 4.367472073101515306, 7.564683531250000925 ) ) ;
#74497=CARTESIAN_POINT ( 'NONE',  ( 129.5000000000000000, 0.000000000000000000, 0.000000000000000000 ) ) ;
#74530=CARTESIAN_POINT ( 'NONE',  ( 187.1302083336747444, -4.367472073101514418, -7.564683531250002702 ) ) ;
#74587=CARTESIAN_POINT ( 'NONE',  ( 104.9410342067506150, 6.602324511409650043, -3.967845207721173661 ) ) ;
#74623=LINE ( 'NONE', #76561, #56290 ) ;
#74661=ORIENTED_EDGE ( 'NONE', *, *, #116320, .F. ) ;
#74815=CARTESIAN_POINT ( 'NONE',  ( 185.7552083336747444, 6.551208109652275624, -3.782341765624998686 ) ) ;
#74847=CARTESIAN_POINT ( 'NONE',  ( 186.6250000000000000, -8.891194145520236347, -1.633285867636356299E-15 ) ) ;
#74878=CARTESIAN_POINT ( 'NONE',  ( 88.00000000000001421, 0.000000000000000000, -8.199999999999999289 ) ) ;
#75033=ORIENTED_EDGE ( 'NONE', *, *, #97705, .T. ) ;
#75060=CARTESIAN_POINT ( 'NONE',  ( 183.9062500006828031, -8.891194145520236347, -1.633285867636356693E-15 ) ) ;
#75069=ORIENTED_EDGE ( 'NONE', *, *, #99768, .T. ) ;
#75118=VERTEX_POINT ( 'NONE', #32796 ) ;
#75174=CARTESIAN_POINT ( 'NONE',  ( 186.7812500006828031, 0.000000000000000000, 7.700000000000000178 ) ) ;
#75202=LINE ( 'NONE', #104021, #49694 ) ;
#75216=CARTESIAN_POINT ( 'NONE',  ( 109.6452891074249720, 6.075908156944702654, -4.732659750966558221 ) ) ;
#75362=FACE_OUTER_BOUND ( 'NONE', #84988, .T. ) ;
#75375=ORIENTED_EDGE ( 'NONE', *, *, #112539, .F. ) ;
#75395=( BOUNDED_CURVE ( )  B_SPLINE_CURVE ( 2, ( #62974, #102886, #70869, #40787, #52503, #32252, #122549 ),
 .UNSPECIFIED., .F., .F. ) 
 B_SPLINE_CURVE_WITH_KNOTS ( ( 3, 2, 2, 3 ),
 ( 0.7857142857142862535, 0.8095238095238102005, 0.8333333333333340365, 0.8571428571428578724 ),
 .UNSPECIFIED. ) 
 CURVE ( )  GEOMETRIC_REPRESENTATION_ITEM ( )  RATIONAL_B_SPLINE_CURVE ( ( 0.9999999999999968914, 0.8660254037844418162, 1.000000000000000000, 0.8660254037844387076, 1.000000000000000000, 0.8660254037844343777, 1.000000000000004441 ) ) 
 REPRESENTATION_ITEM ( '' )  );
#75412=ORIENTED_EDGE ( 'NONE', *, *, #59684, .T. ) ;
#75444=CARTESIAN_POINT ( 'NONE',  ( 185.5468750003414300, -8.734944146203032389, -1.604583208406768146E-15 ) ) ;
#75544=CARTESIAN_POINT ( 'NONE',  ( 184.6666666666666856, -6.668395609140176816, -3.850000000000003642 ) ) ;
#75565=ADVANCED_FACE ( 'NONE', ( #12958, #92845 ), #1861, .F. ) ;
#75685=CARTESIAN_POINT ( 'NONE',  ( 185.1145833340161175, 6.668395609140177704, -3.849999999999998312 ) ) ;
#75733=CARTESIAN_POINT ( 'NONE',  ( 184.3385416670080872, 6.551208109652274736, 3.782341765625001351 ) ) ;
#75801=CARTESIAN_POINT ( 'NONE',  ( 185.7135416670080588, 4.367472073101518859, -7.564683531249999149 ) ) ;
#75805=AXIS2_PLACEMENT_3D ( 'NONE', #14770, #125406, #105769 ) ;
#75825=ORIENTED_EDGE ( 'NONE', *, *, #2523, .F. ) ;
#75924=CARTESIAN_POINT ( 'NONE',  ( 187.0312500006828031, 9.429780353434619030E-16, -7.700000000000000178 ) ) ;
#75936=DIRECTION ( 'NONE',  ( 1.000000000000000000, 0.000000000000000000, 0.000000000000000000 ) ) ;
#75964=EDGE_CURVE ( 'NONE', #115280, #59105, #71583, .T. ) ;
#76006=DIRECTION ( 'NONE',  ( 0.000000000000000000, 0.000000000000000000, -1.000000000000000000 ) ) ;
#76027=DIRECTION ( 'NONE',  ( 0.000000000000000000, 1.000000000000000000, -1.846105847067148761E-16 ) ) ;
#76033=EDGE_CURVE ( 'NONE', #27968, #126401, #27086, .T. ) ;
#76103=CARTESIAN_POINT ( 'NONE',  ( 185.9583333333333428, 4.445597072760117285, 7.699999999999999289 ) ) ;
#76128=VECTOR ( 'NONE', #68560, 1000.000000000000000 ) ;
#76231=CARTESIAN_POINT ( 'NONE',  ( 187.5000000000000000, 0.000000000000000000, 7.700000000000000178 ) ) ;
#76322=PLANE ( 'NONE',  #6621 ) ;
#76355=CARTESIAN_POINT ( 'NONE',  ( 184.5729166673494603, 4.445597072760120838, -7.699999999999998401 ) ) ;
#76366=DIRECTION ( 'NONE',  ( 0.000000000000000000, 1.846105847067148022E-16, -1.000000000000000000 ) ) ;
#76398=CARTESIAN_POINT ( 'NONE',  ( 185.1302083336747160, -4.367472073101514418, -7.564683531250002702 ) ) ;
#76467=CARTESIAN_POINT ( 'NONE',  ( 184.6718750003414016, 9.264065473108010111E-16, -7.564683531250000925 ) ) ;
#76539=CARTESIAN_POINT ( 'NONE',  ( 187.2083333333333712, -4.445597072760123503, -7.699999999999989519 ) ) ;
#76561=CARTESIAN_POINT ( 'NONE',  ( 187.5000000000000000, -1.375000000000000000, 7.576237522675751457 ) ) ;
#76661=ORIENTED_EDGE ( 'NONE', *, *, #34794, .T. ) ;
#76669=ORIENTED_EDGE ( 'NONE', *, *, #86187, .F. ) ;
#76748=CARTESIAN_POINT ( 'NONE',  ( 184.7916666666666856, 4.445597072760120838, -7.699999999999998401 ) ) ;
#76781=CARTESIAN_POINT ( 'NONE',  ( 186.6666666666666856, -6.668395609140176816, -3.850000000000003642 ) ) ;
#76789=LINE ( 'NONE', #98340, #88146 ) ;
#76853=ORIENTED_EDGE ( 'NONE', *, *, #36681, .T. ) ;
#76870=EDGE_CURVE ( 'NONE', #99802, #3837, #38619, .T. ) ;
#76871=ORIENTED_EDGE ( 'NONE', *, *, #70434, .T. ) ;
#76894=DIRECTION ( 'NONE',  ( -1.000000000000000000, 0.000000000000000000, 0.000000000000000000 ) ) ;
#76901=LINE ( 'NONE', #88653, #105399 ) ;
#76990=CARTESIAN_POINT ( 'NONE',  ( 186.5677083336747160, -4.367472073101514418, -7.564683531250002702 ) ) ;
#77037=CARTESIAN_POINT ( 'NONE',  ( 185.7968750003414300, 8.734944146203032389, 5.348610694689227483E-16 ) ) ;
#77053=VERTEX_POINT ( 'NONE', #16827 ) ;
#77108=CARTESIAN_POINT ( 'NONE',  ( 184.4218750003414016, 0.000000000000000000, 7.564683531250000925 ) ) ;
#77327=SURFACE_STYLE_USAGE ( .BOTH. , #9238 ) ;
#77379=DIRECTION ( 'NONE',  ( -1.000000000000000000, -0.000000000000000000, -0.000000000000000000 ) ) ;
#77393=CARTESIAN_POINT ( 'NONE',  ( 186.0416666666666856, -4.445597072760122614, 7.699999999999998401 ) ) ;
#77401=FACE_OUTER_BOUND ( 'NONE', #85778, .T. ) ;
#77438=CYLINDRICAL_SURFACE ( 'NONE', #38459, 5.000000000000004441 ) ;
#77482=CARTESIAN_POINT ( 'NONE',  ( 129.5000000000000000, -1.500000000000000000, -6.000000000000000000 ) ) ;
#77501=EDGE_CURVE ( 'NONE', #7606, #115280, #55350, .T. ) ;
#77589=ADVANCED_FACE ( 'NONE', ( #104445 ), #105740, .F. ) ;
#77621=CARTESIAN_POINT ( 'NONE',  ( 187.3593750003414016, 0.000000000000000000, 7.564683531250000925 ) ) ;
#77691=( BOUNDED_CURVE ( )  B_SPLINE_CURVE ( 2, ( #52962, #43162, #42511, #101416, #102062, #121046, #92896 ),
 .UNSPECIFIED., .F., .F. ) 
 B_SPLINE_CURVE_WITH_KNOTS ( ( 3, 2, 2, 3 ),
 ( 0.9285714285714292693, 0.9523809523809527722, 0.9761904761904763861, 1.000000000000000000 ),
 .UNSPECIFIED. ) 
 CURVE ( )  GEOMETRIC_REPRESENTATION_ITEM ( )  RATIONAL_B_SPLINE_CURVE ( ( 0.9999999999999962252, 0.8660254037844424824, 1.000000000000000000, 0.8660254037844387076, 1.000000000000000000, 0.8660254037844387076, 1.000000000000000000 ) ) 
 REPRESENTATION_ITEM ( '' )  );
#77727=CARTESIAN_POINT ( 'NONE',  ( 184.5885416670080872, -6.551208109652273848, -3.782341765625003571 ) ) ;
#77738=AXIS2_PLACEMENT_3D ( 'NONE', #82145, #59950, #81502 ) ;
#77805=CARTESIAN_POINT ( 'NONE',  ( 187.1249999999999716, -8.891194145520236347, -1.633285867636356299E-15 ) ) ;
#77821=CARTESIAN_POINT ( 'NONE',  ( 187.1510416670080303, 4.367472073101518859, -7.564683531249999149 ) ) ;
#77869=CIRCLE ( 'NONE', #111305, 7.700000000000000178 ) ;
#77951=CARTESIAN_POINT ( 'NONE',  ( 187.5000000000000000, 0.000000000000000000, 7.700000000000000178 ) ) ;
#78001=VECTOR ( 'NONE', #66504, 1000.000000000000000 ) ;
#78034=ORIENTED_EDGE ( 'NONE', *, *, #126217, .F. ) ;
#78035=CARTESIAN_POINT ( 'NONE',  ( 185.1250000000000284, -8.891194145520236347, -1.633285867636356693E-15 ) ) ;
#78083=CARTESIAN_POINT ( 'NONE',  ( 179.5000000000000000, -0.6250000000000000000, 7.634788798650553154 ) ) ;
#78202=DIRECTION ( 'NONE',  ( 0.000000000000000000, 0.000000000000000000, 1.000000000000000000 ) ) ;
#78246=ORIENTED_EDGE ( 'NONE', *, *, #70570, .T. ) ;
#78299=CARTESIAN_POINT ( 'NONE',  ( 186.1510416670080588, 4.367472073101518859, -7.564683531249999149 ) ) ;
#78334=CARTESIAN_POINT ( 'NONE',  ( 187.5000000000000000, 0.000000000000000000, 0.000000000000000000 ) ) ;
#78416=CARTESIAN_POINT ( 'NONE',  ( 184.7552083336747444, 6.551208109652275624, -3.782341765624998686 ) ) ;
#78465=CARTESIAN_POINT ( 'NONE',  ( 112.3162792014981619, 7.273147445303300707, -2.544068225761106472 ) ) ;
#78503=CARTESIAN_POINT ( 'NONE',  ( 187.0260416670080588, -6.551208109652273848, -3.782341765625003571 ) ) ;
#78544=DIRECTION ( 'NONE',  ( 0.000000000000000000, 1.000000000000000000, 0.000000000000000000 ) ) ;
#78577=ORIENTED_EDGE ( 'NONE', *, *, #21838, .F. ) ;
#78700=CARTESIAN_POINT ( 'NONE',  ( 186.4166666666666856, 6.668395609140176816, 3.850000000000000977 ) ) ;
#78789=CARTESIAN_POINT ( 'NONE',  ( 185.1250000000000000, -8.891194145520236347, -1.633285867636356299E-15 ) ) ;
#78847=CARTESIAN_POINT ( 'NONE',  ( 184.0312500006828031, 9.429780353434619030E-16, -7.700000000000000178 ) ) ;
#78940=ADVANCED_BREP_SHAPE_REPRESENTATION ( '', ( #57499, #108296 ), #20574 ) ;
#78941=CARTESIAN_POINT ( 'NONE',  ( 184.9010416670080588, -4.367472073101519747, 7.564683531249999149 ) ) ;
#78974=CARTESIAN_POINT ( 'NONE',  ( 179.5000000000000000, 0.6250000000000000000, 7.634788798650556707 ) ) ;
#79091=VERTEX_POINT ( 'NONE', #91153 ) ;
#79141=CARTESIAN_POINT ( 'NONE',  ( 186.3593750003414016, 0.000000000000000000, 7.564683531250000925 ) ) ;
#79159=CLOSED_SHELL ( 'NONE', ( #35992, #44206, #23962, #71006, #90669, #119020, #60205, #81435, #43519, #91832, #26070, #106782, #34979, #37376, #39327, #33335, #13139, #94184, #100289, #8660, #103003, #48814, #85650, #50480, #122277, #55783, #77589, #1819, #98128, #113920, #47131, #75565, #109141, #23021, #14914, #81885, #33929, #108267, #72146, #69832, #121906, #129240, #66265, #104391, #114709, #35407, #63610, #44718, #56483, #114147, #72726, #57424, #32030, #33949, #88081, #124217, #37942, #42290, #59542, #1226 ) ) ;
#79283=DIRECTION ( 'NONE',  ( 0.000000000000000000, -1.846105847067148022E-16, 1.000000000000000000 ) ) ;
#79351=DIRECTION ( 'NONE',  ( -1.000000000000000000, -0.000000000000000000, -0.000000000000000000 ) ) ;
#79381=CARTESIAN_POINT ( 'NONE',  ( 186.5260416670080588, -6.551208109652273848, -3.782341765625003571 ) ) ;
#79383=CARTESIAN_POINT ( 'NONE',  ( 103.6750765693973761, 8.328912879160041527, 2.529530674324913964 ) ) ;
#79484=CARTESIAN_POINT ( 'NONE',  ( 184.1145833340161175, 6.668395609140177704, -3.849999999999998312 ) ) ;
#79494=DIRECTION ( 'NONE',  ( 0.000000000000000000, 0.000000000000000000, 1.000000000000000000 ) ) ;
#79544=ORIENTED_EDGE ( 'NONE', *, *, #54408, .T. ) ;
#79576=CARTESIAN_POINT ( 'NONE',  ( 185.2760416670080588, 6.551208109652274736, 3.782341765625001351 ) ) ;
#79673=CARTESIAN_POINT ( 'NONE',  ( 179.5000000000000000, -1.375000000000002442, 6.000000000000000000 ) ) ;
#79766=CARTESIAN_POINT ( 'NONE',  ( 185.7343750003414016, 8.734944146203032389, 5.348610694689227483E-16 ) ) ;
#79831=PLANE ( 'NONE',  #107496 ) ;
#79839=DIRECTION ( 'NONE',  ( 0.000000000000000000, -0.000000000000000000, -1.000000000000000000 ) ) ;
#79874=VERTEX_POINT ( 'NONE', #97274 ) ;
#79882=ORIENTED_EDGE ( 'NONE', *, *, #99658, .F. ) ;
#79990=AXIS2_PLACEMENT_3D ( 'NONE', #1865, #62745, #111158 ) ;
#80059=VERTEX_POINT ( 'NONE', #105663 ) ;
#80060=VECTOR ( 'NONE', #73727, 1000.000000000000000 ) ;
#80066=DIRECTION ( 'NONE',  ( 0.000000000000000000, -1.846105847067148515E-16, -1.000000000000000000 ) ) ;
#80186=VERTEX_POINT ( 'NONE', #42898 ) ;
#80223=CARTESIAN_POINT ( 'NONE',  ( 185.3177083336747160, 4.367472073101515306, 7.564683531250000925 ) ) ;
#80320=ORIENTED_EDGE ( 'NONE', *, *, #58862, .F. ) ;
#80357=VECTOR ( 'NONE', #20051, 1000.000000000000000 ) ;
#80425=CARTESIAN_POINT ( 'NONE',  ( 187.3177083336747444, 4.367472073101515306, 7.564683531250000925 ) ) ;
#80456=EDGE_CURVE ( 'NONE', #84030, #60931, #59148, .T. ) ;
#80530=CARTESIAN_POINT ( 'NONE',  ( 184.7812500006828031, 0.000000000000000000, 7.700000000000000178 ) ) ;
#80550=VECTOR ( 'NONE', #81393, 1000.000000000000000 ) ;
#80553=CARTESIAN_POINT ( 'NONE',  ( 104.9453507214960695, 6.600323588196552294, 3.971150466560552150 ) ) ;
#80556=ORIENTED_EDGE ( 'NONE', *, *, #63013, .T. ) ;
#80672=CARTESIAN_POINT ( 'NONE',  ( 104.9394650928313553, 7.745629575256785415, 3.967022963969182747 ) ) ;
#80679=ORIENTED_EDGE ( 'NONE', *, *, #63162, .T. ) ;
#80718=DIRECTION ( 'NONE',  ( 1.000000000000000000, 0.000000000000000000, 0.000000000000000000 ) ) ;
#80750=CARTESIAN_POINT ( 'NONE',  ( 112.7324313128099220, 8.548364151789236587, -1.646368127929983327 ) ) ;
#80755=ORIENTED_EDGE ( 'NONE', *, *, #13761, .T. ) ;
#80783=CARTESIAN_POINT ( 'NONE',  ( 187.3802083336747444, 4.367472073101515306, 7.564683531250000925 ) ) ;
#80794=CARTESIAN_POINT ( 'NONE',  ( 179.5000000000000000, 1.375000000000000000, 7.634788798650556707 ) ) ;
#80868=CARTESIAN_POINT ( 'NONE',  ( 183.9427083336747160, -6.551208109652278289, 3.782341765624995134 ) ) ;
#80875=LINE ( 'NONE', #2955, #86051 ) ;
#80901=CARTESIAN_POINT ( 'NONE',  ( 184.7812500006828031, 0.000000000000000000, 7.700000000000000178 ) ) ;
#81040=PLANE ( 'NONE',  #3588 ) ;
#81042=PLANE ( 'NONE',  #107967 ) ;
#81068=CARTESIAN_POINT ( 'NONE',  ( 186.6718750003414016, 9.264065473108010111E-16, -7.564683531250000925 ) ) ;
#81080=ORIENTED_EDGE ( 'NONE', *, *, #75964, .F. ) ;
#81142=CARTESIAN_POINT ( 'NONE',  ( 183.8203125005121024, 0.000000000000000000, 7.632341765625000107 ) ) ;
#81186=EDGE_CURVE ( 'NONE', #16632, #4736, #25480, .T. ) ;
#81195=ORIENTED_EDGE ( 'NONE', *, *, #8037, .F. ) ;
#81215=( GEOMETRIC_REPRESENTATION_CONTEXT ( 3 ) GLOBAL_UNCERTAINTY_ASSIGNED_CONTEXT ( ( #19173 ) ) GLOBAL_UNIT_ASSIGNED_CONTEXT ( ( #127086, #89723, #37417 ) ) REPRESENTATION_CONTEXT ( 'NONE', 'WORKASPACE' ) );
#81309=CARTESIAN_POINT ( 'NONE',  ( 184.5260416670080588, -6.551208109652273848, -3.782341765625003571 ) ) ;
#81316=AXIS2_PLACEMENT_3D ( 'NONE', #91969, #109682, #122720 ) ;
#81393=DIRECTION ( 'NONE',  ( -1.000000000000000000, 0.000000000000000000, 0.000000000000000000 ) ) ;
#81397=CARTESIAN_POINT ( 'NONE',  ( 110.5209590753869406, 7.548722077129768060, 4.329966018956735496 ) ) ;
#81431=PLANE ( 'NONE',  #84828 ) ;
#81435=ADVANCED_FACE ( 'NONE', ( #83630 ), #111802, .F. ) ;
#81502=DIRECTION ( 'NONE',  ( 0.000000000000000000, 0.000000000000000000, -1.000000000000000000 ) ) ;
#81560=DIRECTION ( 'NONE',  ( 0.000000000000000000, 0.000000000000000000, -1.000000000000000000 ) ) ;
#81585=VECTOR ( 'NONE', #33021, 1000.000000000000000 ) ;
#81590=CARTESIAN_POINT ( 'NONE',  ( 186.4895833340161460, -4.445597072760135937, -7.699999999999966427 ) ) ;
#81594=EDGE_CURVE ( 'NONE', #29124, #84030, #7620, .T. ) ;
#81609=LINE ( 'NONE', #13507, #120293 ) ;
#81693=CARTESIAN_POINT ( 'NONE',  ( 184.1093750003413732, 9.264065473108010111E-16, -7.564683531250000925 ) ) ;
#81722=ORIENTED_EDGE ( 'NONE', *, *, #89301, .F. ) ;
#81818=CARTESIAN_POINT ( 'NONE',  ( 102.9915580679601135, 7.705489964099487388, 0.005789880036570591894 ) ) ;
#81885=ADVANCED_FACE ( 'NONE', ( #93772 ), #34590, .T. ) ;
#81892=( BOUNDED_CURVE ( )  B_SPLINE_CURVE ( 2, ( #107701, #18015, #85475, #8196, #117479, #47495, #116857 ),
 .UNSPECIFIED., .F., .F. ) 
 B_SPLINE_CURVE_WITH_KNOTS ( ( 3, 2, 2, 3 ),
 ( 0.7142857142857148567, 0.7380952380952386926, 0.7619047619047624176, 0.7857142857142862535 ),
 .UNSPECIFIED. ) 
 CURVE ( )  GEOMETRIC_REPRESENTATION_ITEM ( )  RATIONAL_B_SPLINE_CURVE ( ( 0.9999999999999968914, 0.8660254037844418162, 1.000000000000000000, 0.8660254037844387076, 1.000000000000000000, 0.8660254037844355990, 1.000000000000003109 ) ) 
 REPRESENTATION_ITEM ( '' )  );
#81931=CARTESIAN_POINT ( 'NONE',  ( 184.0260416670080588, -6.551208109652273848, -3.782341765625003571 ) ) ;
#81993=AXIS2_PLACEMENT_3D ( 'NONE', #62613, #60682, #33154 ) ;
#82046=CARTESIAN_POINT ( 'NONE',  ( 186.4635416670080872, -4.367472073101519747, 7.564683531249999149 ) ) ;
#82062=ORIENTED_EDGE ( 'NONE', *, *, #76033, .T. ) ;
#82087=AXIS2_PLACEMENT_3D ( 'NONE', #44057, #84632, #102970 ) ;
#82107=DIRECTION ( 'NONE',  ( 0.000000000000000000, -1.000000000000000000, -0.000000000000000000 ) ) ;
#82145=CARTESIAN_POINT ( 'NONE',  ( 129.5000000000000000, 0.000000000000000000, 0.000000000000000000 ) ) ;
#82258=ORIENTED_EDGE ( 'NONE', *, *, #115339, .F. ) ;
#82268=FACE_OUTER_BOUND ( 'NONE', #5017, .T. ) ;
#82271=CYLINDRICAL_SURFACE ( 'NONE', #65803, 7.700000000000000178 ) ;
#82291=DIRECTION ( 'NONE',  ( -1.000000000000000000, 0.000000000000000000, 0.000000000000000000 ) ) ;
#82357=EDGE_CURVE ( 'NONE', #43167, #80186, #46753, .T. ) ;
#82365=CARTESIAN_POINT ( 'NONE',  ( 184.4843750003414016, -8.734944146203032389, -1.604583208406768146E-15 ) ) ;
#82436=CARTESIAN_POINT ( 'NONE',  ( 187.2135416670080303, 4.367472073101518859, -7.564683531249999149 ) ) ;
#82501=CARTESIAN_POINT ( 'NONE',  ( 185.0312500006828031, 9.429780353434619030E-16, -7.700000000000000178 ) ) ;
#82545=CARTESIAN_POINT ( 'NONE',  ( 187.1145833340161175, 6.668395609140177704, -3.849999999999998312 ) ) ;
#82603=CARTESIAN_POINT ( 'NONE',  ( 185.0260416670080588, -6.551208109652273848, -3.782341765625003571 ) ) ;
#82646=EDGE_LOOP ( 'NONE', ( #106150, #70818, #74282, #13228 ) ) ;
#82659=EDGE_CURVE ( 'NONE', #103176, #69132, #90880, .T. ) ;
#82667=CARTESIAN_POINT ( 'NONE',  ( 185.1145833340161175, 6.668395609140177704, -3.849999999999998312 ) ) ;
#82675=( LENGTH_UNIT ( ) NAMED_UNIT ( * ) SI_UNIT ( .MILLI., .METRE. ) );
#82719=CARTESIAN_POINT ( 'NONE',  ( 187.1666666666666856, -6.668395609140176816, -3.850000000000003642 ) ) ;
#83005=CARTESIAN_POINT ( 'NONE',  ( 184.6927083336747160, 6.551208109652275624, -3.782341765624998686 ) ) ;
#83147=DIRECTION ( 'NONE',  ( 0.000000000000000000, 1.000000000000000000, 0.000000000000000000 ) ) ;
#83148=CARTESIAN_POINT ( 'NONE',  ( 127.5000000000000000, 1.500000000000000000, -2.598076211353316900 ) ) ;
#83231=EDGE_CURVE ( 'NONE', #55407, #23165, #7448, .T. ) ;
#83249=CARTESIAN_POINT ( 'NONE',  ( 184.1927083336747160, 6.551208109652275624, -3.782341765624998686 ) ) ;
#83312=VERTEX_POINT ( 'NONE', #31596 ) ;
#83356=CARTESIAN_POINT ( 'NONE',  ( 185.8385416670080872, 6.551208109652274736, 3.782341765625001351 ) ) ;
#83357=DIRECTION ( 'NONE',  ( -1.000000000000000000, -0.000000000000000000, -0.000000000000000000 ) ) ;
#83388=AXIS2_PLACEMENT_3D ( 'NONE', #74878, #84034, #112872 ) ;
#83418=DIRECTION ( 'NONE',  ( 0.000000000000000000, 0.000000000000000000, -1.000000000000000000 ) ) ;
#83481=DIRECTION ( 'NONE',  ( 1.000000000000000000, 0.000000000000000000, -0.000000000000000000 ) ) ;
#83514=DIRECTION ( 'NONE',  ( -1.000000000000000000, -0.000000000000000000, -0.000000000000000000 ) ) ;
#83536=CARTESIAN_POINT ( 'NONE',  ( 187.2500000000000000, 9.429780353434619030E-16, -7.700000000000000178 ) ) ;
#83551=EDGE_CURVE ( 'NONE', #80186, #127679, #16433, .T. ) ;
#83599=CARTESIAN_POINT ( 'NONE',  ( 186.9479166673494603, -6.668395609140176816, -3.850000000000003642 ) ) ;
#83630=FACE_OUTER_BOUND ( 'NONE', #55710, .T. ) ;
#83643=CARTESIAN_POINT ( 'NONE',  ( 186.1302083336747444, -4.367472073101514418, -7.564683531250002702 ) ) ;
#83769=CARTESIAN_POINT ( 'NONE',  ( 187.3203125005121024, 0.000000000000000000, 7.632341765625000107 ) ) ;
#83868=CARTESIAN_POINT ( 'NONE',  ( 185.7760416670080588, 6.551208109652274736, 3.782341765625001351 ) ) ;
#83961=VECTOR ( 'NONE', #44895, 1000.000000000000000 ) ;
#83962=AXIS2_PLACEMENT_3D ( 'NONE', #56481, #68888, #96404 ) ;
#83972=CARTESIAN_POINT ( 'NONE',  ( 185.5885416670080872, -6.551208109652273848, -3.782341765625003571 ) ) ;
#84030=VERTEX_POINT ( 'NONE', #107258 ) ;
#84034=DIRECTION ( 'NONE',  ( 0.000000000000000000, -1.000000000000000000, 0.000000000000000000 ) ) ;
#84093=AXIS2_PLACEMENT_3D ( 'NONE', #43462, #3521, #95127 ) ;
#84184=CARTESIAN_POINT ( 'NONE',  ( 184.2500000000000000, 9.429780353434619030E-16, -7.700000000000000178 ) ) ;
#84269=CARTESIAN_POINT ( 'NONE',  ( 184.5468750003414300, -8.734944146203032389, -1.604583208406768146E-15 ) ) ;
#84347=CARTESIAN_POINT ( 'NONE',  ( 186.7968750003414300, 8.734944146203032389, 5.348610694689227483E-16 ) ) ;
#84403=ORIENTED_EDGE ( 'NONE', *, *, #63330, .F. ) ;
#84474=ORIENTED_EDGE ( 'NONE', *, *, #56849, .F. ) ;
#84488=EDGE_LOOP ( 'NONE', ( #90625, #71095, #28681, #79882 ) ) ;
#84519=ORIENTED_EDGE ( 'NONE', *, *, #39747, .F. ) ;
#84584=( BOUNDED_SURFACE ( )  B_SPLINE_SURFACE ( 1, 2, ( 
 ( #110515, #80425, #28092, #38580, #50970, #77821, #120347, #68008, #78503, #127582, #117734, #109212, #69283, #60778, #89592, #129543, #548, #58215, #39235, #8432, #118397, #37905, #40513, #28747, #79141, #107934, #98110, #19558, #9089, #48375, #60153, #90211, #88271, #108583, #119054, #18900, #128242, #109880, #58841, #79766, #98749, #9739, #49041, #119680, #59516, #30688, #99426, #30038, #100680, #100058, #29394, #10382, #69955, #20207, #70595, #11008, #90874, #62720, #14232, #111137, #1204, #103283, #13588, #51610, #83005, #113750, #101993, #92823, #41802, #82365, #102618, #33886, #43096, #71895, #22162, #122925, #12938, #24075, #81693, #12306, #61437, #32637, #73803, #43735, #121612 ),
 ( #21491, #22804, #11667, #31972, #41156, #120982, #62074, #42434, #33268, #52248, #122284, #113087, #63994, #103921, #101351, #92157, #123542, #73173, #81068, #72539, #23412, #31331, #71228, #53540, #91524, #2475, #3151, #1841, #111817, #112464, #63352, #83643, #52889, #93453, #3786, #46277, #27279, #15520, #37122, #77037, #5061, #14858, #26650, #6327, #96651, #65916, #36489, #54803, #67177, #24719, #55466, #45009, #86184, #35195, #107122, #76398, #26011, #116297, #105851, #115656, #56718, #74461, #125486, #86848, #95388, #66556, #5699, #116939, #6974, #84269, #94734, #54182, #4393, #35823, #75733, #94098, #16151, #56094, #46948, #114371, #45655, #64632, #84919, #44345, #126786 ) ),
 .UNSPECIFIED., .F., .F., .F. ) 
 B_SPLINE_SURFACE_WITH_KNOTS ( ( 2, 2 ),
 ( 3, 2, 2, 2, 2, 2, 2, 2, 2, 2, 2, 2, 2, 2, 2, 2, 2, 2, 2, 2, 2, 2, 2, 2, 2, 2, 2, 2, 2, 2, 2, 2, 2, 2, 2, 2, 2, 2, 2, 2, 2, 2, 3 ),
 ( 0.000000000000000000, 1.000000000000000000 ),
 ( 0.000000000000000000, 0.02380952380952380820, 0.04761904761904761640, 0.07142857142857142461, 0.09523809523809523281, 0.1190476190476190410, 0.1428571428571428492, 0.1666666666666666574, 0.1904761904761904656, 0.2142857142857142738, 0.2380952380952380820, 0.2619047619047619180, 0.2857142857142856984, 0.3095238095238095344, 0.3333333333333333148, 0.3571428571428571508, 0.3809523809523809312, 0.4047619047619047672, 0.4285714285714285476, 0.4523809523809523836, 0.4761904761904761640, 0.5000000000000000000, 0.5238095238095238360, 0.5476190476190476719, 0.5714285714285713969, 0.5952380952380952328, 0.6190476190476190688, 0.6428571428571429047, 0.6666666666666666297, 0.6904761904761904656, 0.7142857142857143016, 0.7380952380952381375, 0.7619047619047618625, 0.7857142857142856984, 0.8095238095238095344, 0.8333333333333333703, 0.8571428571428570953, 0.8809523809523809312, 0.9047619047619047672, 0.9285714285714286031, 0.9523809523809523281, 0.9761904761904761640, 1.000000000000000000 ),
 .UNSPECIFIED. ) 
 GEOMETRIC_REPRESENTATION_ITEM ( )  RATIONAL_B_SPLINE_SURFACE ( (
 ( 1.000000000000000000, 0.8660254037844387076, 1.000000000000000000, 0.8660254037844387076, 1.000000000000000000, 0.8660254037844387076, 1.000000000000000000, 0.8660254037844387076, 1.000000000000000000, 0.8660254037844387076, 1.000000000000000000, 0.8660254037844387076, 1.000000000000000000, 0.8660254037844387076, 1.000000000000000000, 0.8660254037844387076, 1.000000000000000000, 0.8660254037844387076, 1.000000000000000000, 0.8660254037844387076, 1.000000000000000000, 0.8660254037844387076, 1.000000000000000000, 0.8660254037844387076, 1.000000000000000000, 0.8660254037844387076, 1.000000000000000000, 0.8660254037844387076, 1.000000000000000000, 0.8660254037844387076, 1.000000000000000000, 0.8660254037844387076, 1.000000000000000000, 0.8660254037844387076, 1.000000000000000000, 0.8660254037844387076, 1.000000000000000000, 0.8660254037844387076, 1.000000000000000000, 0.8660254037844387076, 1.000000000000000000, 0.8660254037844387076, 1.000000000000000000, 0.8660254037844387076, 1.000000000000000000, 0.8660254037844387076, 1.000000000000000000, 0.8660254037844387076, 1.000000000000000000, 0.8660254037844387076, 1.000000000000000000, 0.8660254037844387076, 1.000000000000000000, 0.8660254037844387076, 1.000000000000000000, 0.8660254037844387076, 1.000000000000000000, 0.8660254037844387076, 1.000000000000000000, 0.8660254037844387076, 1.000000000000000000, 0.8660254037844387076, 1.000000000000000000, 0.8660254037844387076, 1.000000000000000000, 0.8660254037844387076, 1.000000000000000000, 0.8660254037844387076, 1.000000000000000000, 0.8660254037844387076, 1.000000000000000000, 0.8660254037844387076, 1.000000000000000000, 0.8660254037844387076, 1.000000000000000000, 0.8660254037844387076, 1.000000000000000000, 0.8660254037844387076, 1.000000000000000000, 0.8660254037844387076, 1.000000000000000000, 0.8660254037844387076, 1.000000000000000000, 0.8660254037844387076, 1.000000000000000000),
 ( 1.000000000000000000, 0.8660254037844387076, 1.000000000000000000, 0.8660254037844387076, 1.000000000000000000, 0.8660254037844387076, 1.000000000000000000, 0.8660254037844387076, 1.000000000000000000, 0.8660254037844387076, 1.000000000000000000, 0.8660254037844387076, 1.000000000000000000, 0.8660254037844387076, 1.000000000000000000, 0.8660254037844387076, 1.000000000000000000, 0.8660254037844387076, 1.000000000000000000, 0.8660254037844387076, 1.000000000000000000, 0.8660254037844387076, 1.000000000000000000, 0.8660254037844387076, 1.000000000000000000, 0.8660254037844387076, 1.000000000000000000, 0.8660254037844387076, 1.000000000000000000, 0.8660254037844387076, 1.000000000000000000, 0.8660254037844387076, 1.000000000000000000, 0.8660254037844387076, 1.000000000000000000, 0.8660254037844387076, 1.000000000000000000, 0.8660254037844387076, 1.000000000000000000, 0.8660254037844387076, 1.000000000000000000, 0.8660254037844387076, 1.000000000000000000, 0.8660254037844387076, 1.000000000000000000, 0.8660254037844387076, 1.000000000000000000, 0.8660254037844387076, 1.000000000000000000, 0.8660254037844387076, 1.000000000000000000, 0.8660254037844387076, 1.000000000000000000, 0.8660254037844387076, 1.000000000000000000, 0.8660254037844387076, 1.000000000000000000, 0.8660254037844387076, 1.000000000000000000, 0.8660254037844387076, 1.000000000000000000, 0.8660254037844387076, 1.000000000000000000, 0.8660254037844387076, 1.000000000000000000, 0.8660254037844387076, 1.000000000000000000, 0.8660254037844387076, 1.000000000000000000, 0.8660254037844387076, 1.000000000000000000, 0.8660254037844387076, 1.000000000000000000, 0.8660254037844387076, 1.000000000000000000, 0.8660254037844387076, 1.000000000000000000, 0.8660254037844387076, 1.000000000000000000, 0.8660254037844387076, 1.000000000000000000, 0.8660254037844387076, 1.000000000000000000, 0.8660254037844387076, 1.000000000000000000) ) ) 
 REPRESENTATION_ITEM ( '' )  SURFACE ( )  );
#84632=DIRECTION ( 'NONE',  ( 0.000000000000000000, -1.000000000000000000, 0.000000000000000000 ) ) ;
#84634=CARTESIAN_POINT ( 'NONE',  ( 185.2135416670080872, 4.367472073101518859, -7.564683531249999149 ) ) ;
#84677=FACE_OUTER_BOUND ( 'NONE', #61097, .T. ) ;
#84828=AXIS2_PLACEMENT_3D ( 'NONE', #80794, #29742, #10102 ) ;
#84873=CARTESIAN_POINT ( 'NONE',  ( 184.6145833340161175, 6.668395609140177704, -3.849999999999998312 ) ) ;
#84884=CARTESIAN_POINT ( 'NONE',  ( 187.3906250003414016, 0.000000000000000000, 7.564683531250000925 ) ) ;
#84919=CARTESIAN_POINT ( 'NONE',  ( 184.0052083336747160, -6.551208109652278289, 3.782341765624995134 ) ) ;
#84988=EDGE_LOOP ( 'NONE', ( #34473, #38393, #65481, #106456 ) ) ;
#85065=EDGE_CURVE ( 'NONE', #92765, #90185, #62222, .T. ) ;
#85141=AXIS2_PLACEMENT_3D ( 'NONE', #67372, #75936, #5891 ) ;
#85271=CARTESIAN_POINT ( 'NONE',  ( 183.9218750003414016, 0.000000000000000000, 7.564683531250000925 ) ) ;
#85384=DIRECTION ( 'NONE',  ( 0.000000000000000000, 0.000000000000000000, -1.000000000000000000 ) ) ;
#85475=CARTESIAN_POINT ( 'NONE',  ( 184.9166666666666856, 6.668395609140176816, 3.850000000000000977 ) ) ;
#85520=CARTESIAN_POINT ( 'NONE',  ( 184.8229166673494603, -4.445597072760122614, 7.699999999999998401 ) ) ;
#85544=ORIENTED_EDGE ( 'NONE', *, *, #28022, .F. ) ;
#85585=ORIENTED_EDGE ( 'NONE', *, *, #13761, .F. ) ;
#85596=ORIENTED_EDGE ( 'NONE', *, *, #76870, .T. ) ;
#85617=VERTEX_POINT ( 'NONE', #45000 ) ;
#85630=CARTESIAN_POINT ( 'NONE',  ( 185.2135416670080588, 4.367472073101518859, -7.564683531249999149 ) ) ;
#85650=ADVANCED_FACE ( 'NONE', ( #54172 ), #35187, .F. ) ;
#85694=DIRECTION ( 'NONE',  ( 1.000000000000000000, 0.000000000000000000, 0.000000000000000000 ) ) ;
#85743=ORIENTED_EDGE ( 'NONE', *, *, #50674, .T. ) ;
#85778=EDGE_LOOP ( 'NONE', ( #35646, #57685, #3736, #92459 ) ) ;
#85826=DIRECTION ( 'NONE',  ( -1.000000000000000000, -0.000000000000000000, -0.000000000000000000 ) ) ;
#85845=AXIS2_PLACEMENT_3D ( 'NONE', #100140, #10456, #79839 ) ;
#85903=CARTESIAN_POINT ( 'NONE',  ( 185.4166666666666856, 6.668395609140176816, 3.850000000000000977 ) ) ;
#85961=CIRCLE ( 'NONE', #54660, 7.700000000000000178 ) ;
#85963=VERTEX_POINT ( 'NONE', #80901 ) ;
#86004=FACE_OUTER_BOUND ( 'NONE', #72649, .T. ) ;
#86051=VECTOR ( 'NONE', #21291, 1000.000000000000000 ) ;
#86071=VERTEX_POINT ( 'NONE', #32473 ) ;
#86088=( BOUNDED_CURVE ( )  B_SPLINE_CURVE ( 2, ( #30182, #695, #118533, #8566, #68799, #19706, #40001 ),
 .UNSPECIFIED., .F., .F. ) 
 B_SPLINE_CURVE_WITH_KNOTS ( ( 3, 2, 2, 3 ),
 ( 0.4285714285714289362, 0.4523809523809527722, 0.4761904761904766081, 0.5000000000000004441 ),
 .UNSPECIFIED. ) 
 CURVE ( )  GEOMETRIC_REPRESENTATION_ITEM ( )  RATIONAL_B_SPLINE_CURVE ( ( 0.9999999999999977796, 0.8660254037844409281, 1.000000000000000000, 0.8660254037844387076, 1.000000000000000000, 0.8660254037844361541, 1.000000000000002442 ) ) 
 REPRESENTATION_ITEM ( '' )  );
#86139=CARTESIAN_POINT ( 'NONE',  ( 184.3645833340161175, -6.668395609140180369, 3.849999999999994760 ) ) ;
#86184=CARTESIAN_POINT ( 'NONE',  ( 185.2552083336747444, 6.551208109652275624, -3.782341765624998686 ) ) ;
#86187=EDGE_CURVE ( 'NONE', #85617, #14892, #107624, .T. ) ;
#86258=CARTESIAN_POINT ( 'NONE',  ( 185.5885416670080872, -6.551208109652273848, -3.782341765625003571 ) ) ;
#86273=AXIS2_PLACEMENT_3D ( 'NONE', #54476, #52551, #45322 ) ;
#86308=ORIENTED_EDGE ( 'NONE', *, *, #21604, .F. ) ;
#86558=CARTESIAN_POINT ( 'NONE',  ( 185.1666666666666856, -6.668395609140176816, -3.850000000000003642 ) ) ;
#86612=EDGE_CURVE ( 'NONE', #59835, #50117, #23583, .T. ) ;
#86637=EDGE_CURVE ( 'NONE', #51195, #13525, #74623, .T. ) ;
#86682=CARTESIAN_POINT ( 'NONE',  ( 186.2083333333333428, -4.445597072760145707, -7.699999999999951328 ) ) ;
#86735=CARTESIAN_POINT ( 'NONE',  ( 187.5000000000000000, 0.000000000000000000, 0.000000000000000000 ) ) ;
#86805=CARTESIAN_POINT ( 'NONE',  ( 186.6093750003414016, 9.264065473108010111E-16, -7.564683531250000925 ) ) ;
#86827=CIRCLE ( 'NONE', #72185, 7.700000000000000178 ) ;
#86848=CARTESIAN_POINT ( 'NONE',  ( 184.7968750003414016, 8.734944146203032389, 5.348610694689227483E-16 ) ) ;
#86875=VERTEX_POINT ( 'NONE', #60786 ) ;
#86901=ORIENTED_EDGE ( 'NONE', *, *, #31260, .T. ) ;
#86913=CARTESIAN_POINT ( 'NONE',  ( 184.5052083336747444, -6.551208109652278289, 3.782341765624995134 ) ) ;
#87072=CARTESIAN_POINT ( 'NONE',  ( 87.50000000000001421, 0.000000000000000000, 0.000000000000000000 ) ) ;
#87197=CARTESIAN_POINT ( 'NONE',  ( 185.0416666666666856, -4.445597072760122614, 7.699999999999998401 ) ) ;
#87337=EDGE_LOOP ( 'NONE', ( #17345, #78577, #42242, #99948, #14725, #11235, #55765 ) ) ;
#87346=LINE ( 'NONE', #127301, #34312 ) ;
#87441=CARTESIAN_POINT ( 'NONE',  ( 186.3593750003414016, 0.000000000000000000, 7.564683531250000925 ) ) ;
#87477=CIRCLE ( 'NONE', #83388, 0.5000000000000004441 ) ;
#87556=CARTESIAN_POINT ( 'NONE',  ( 185.5468750003414300, -8.734944146203032389, -1.604583208406767949E-15 ) ) ;
#87595=ORIENTED_EDGE ( 'NONE', *, *, #4467, .F. ) ;
#87636=LINE ( 'NONE', #98743, #44542 ) ;
#87695=ORIENTED_EDGE ( 'NONE', *, *, #83231, .F. ) ;
#87839=CARTESIAN_POINT ( 'NONE',  ( 186.2500000000000000, 9.429780353434619030E-16, -7.700000000000000178 ) ) ;
#87952=CARTESIAN_POINT ( 'NONE',  ( 111.7561744588909676, 8.047232822298814980, -3.315531987436182604 ) ) ;
#88067=CARTESIAN_POINT ( 'NONE',  ( 186.1093750003413732, 9.264065473108010111E-16, -7.564683531250000925 ) ) ;
#88081=ADVANCED_FACE ( 'NONE', ( #101822 ), #2977, .F. ) ;
#88086=AXIS2_PLACEMENT_3D ( 'NONE', #53607, #52961, #15591 ) ;
#88137=EDGE_CURVE ( 'NONE', #38386, #100714, #50968, .T. ) ;
#88139=CARTESIAN_POINT ( 'NONE',  ( 185.3750000000000000, 8.891194145520236347, 5.444286225454521982E-16 ) ) ;
#88146=VECTOR ( 'NONE', #116057, 1000.000000000000000 ) ;
#88183=LINE ( 'NONE', #59427, #32212 ) ;
#88204=DIRECTION ( 'NONE',  ( -1.000000000000000000, -0.000000000000000000, -0.000000000000000000 ) ) ;
#88229=CARTESIAN_POINT ( 'NONE',  ( 112.8336731274835643, 7.592877920657278068, 1.321915336562208276 ) ) ;
#88257=PRODUCT_CONTEXT ( 'NONE', #31330, 'mechanical' ) ;
#88271=CARTESIAN_POINT ( 'NONE',  ( 186.0260416670080588, -6.551208109652273848, -3.782341765625003571 ) ) ;
#88395=DIRECTION ( 'NONE',  ( 0.000000000000000000, 0.000000000000000000, 1.000000000000000000 ) ) ;
#88420=LINE ( 'NONE', #49181, #21405 ) ;
#88428=PRODUCT_DEFINITION ( 'UNKNOWN', '', #25460, #116111 ) ;
#88490=CARTESIAN_POINT ( 'NONE',  ( 184.4166666666666856, 6.668395609140176816, 3.850000000000000977 ) ) ;
#88512=CARTESIAN_POINT ( 'NONE',  ( 185.2812500006828031, 0.000000000000000000, 7.700000000000000178 ) ) ;
#88539=CARTESIAN_POINT ( 'NONE',  ( 104.0382667140819990, 8.146203828384356527, -3.067605667726266194 ) ) ;
#88587=CARTESIAN_POINT ( 'NONE',  ( 185.0833333333333144, -6.668395609140180369, 3.849999999999994760 ) ) ;
#88623=CARTESIAN_POINT ( 'NONE',  ( 111.0559149355470936, 7.743809555462367378, 3.970544583781440373 ) ) ;
#88653=CARTESIAN_POINT ( 'NONE',  ( 127.5000000000000000, 1.500000000000000000, 6.000000000000000000 ) ) ;
#88717=EDGE_LOOP ( 'NONE', ( #8505, #45248, #63745 ) ) ;
#88746=CARTESIAN_POINT ( 'NONE',  ( 184.4843750003414016, -8.734944146203032389, -1.604583208406768146E-15 ) ) ;
#88866=ORIENTED_EDGE ( 'NONE', *, *, #104968, .T. ) ;
#88899=LINE ( 'NONE', #71182, #13834 ) ;
#88911=CARTESIAN_POINT ( 'NONE',  ( 112.8293778049783924, 7.590139747709709006, -1.337168253467446277 ) ) ;
#89082=ORIENTED_EDGE ( 'NONE', *, *, #223, .F. ) ;
#89156=LINE ( 'NONE', #1410, #31002 ) ;
#89158=ORIENTED_EDGE ( 'NONE', *, *, #14729, .F. ) ;
#89192=CARTESIAN_POINT ( 'NONE',  ( 105.4784750942634588, 7.548935851765135929, -4.329562946656615452 ) ) ;
#89234=AXIS2_PLACEMENT_3D ( 'NONE', #87072, #18975, #56956 ) ;
#89295=CARTESIAN_POINT ( 'NONE',  ( 187.0885416670080872, -6.551208109652273848, -3.782341765625003571 ) ) ;
#89301=EDGE_CURVE ( 'NONE', #90185, #101564, #112311, .T. ) ;
#89344=AXIS2_PLACEMENT_3D ( 'NONE', #107251, #99381, #39189 ) ;
#89393=CARTESIAN_POINT ( 'NONE',  ( 184.9843750003414016, -8.734944146203032389, -1.604583208406768146E-15 ) ) ;
#89535=CARTESIAN_POINT ( 'NONE',  ( 179.5000000000000000, -0.6250000000000025535, -6.000000000000000888 ) ) ;
#89547=CARTESIAN_POINT ( 'NONE',  ( 111.0560539298719647, 6.600968029026939021, 3.970093675385399479 ) ) ;
#89592=CARTESIAN_POINT ( 'NONE',  ( 186.7760416670080588, 6.551208109652274736, 3.782341765625001351 ) ) ;
#89613=CARTESIAN_POINT ( 'NONE',  ( 127.5000000000000000, 1.500000000000000000, 2.598076211353316900 ) ) ;
#89625=ORIENTED_EDGE ( 'NONE', *, *, #20761, .F. ) ;
#89648=CARTESIAN_POINT ( 'NONE',  ( 187.4583333333333428, 4.445597072760117285, 7.700000000000001066 ) ) ;
#89723=( NAMED_UNIT ( * ) PLANE_ANGLE_UNIT ( ) SI_UNIT ( $, .RADIAN. ) );
#89728=FACE_OUTER_BOUND ( 'NONE', #14268, .T. ) ;
#89830=CARTESIAN_POINT ( 'NONE',  ( 103.0416006710161554, 8.676147590107849084, -0.6650176703920132049 ) ) ;
#89846=CARTESIAN_POINT ( 'NONE',  ( 187.5000000000000000, -1.375000000000002442, -7.576237522675751457 ) ) ;
#89864=UNCERTAINTY_MEASURE_WITH_UNIT (LENGTH_MEASURE( 1.000000000000000082E-05 ), #26307, 'distance_accuracy_value', 'NONE');
#89932=CARTESIAN_POINT ( 'NONE',  ( 187.2552083336747444, 6.551208109652275624, -3.782341765624998686 ) ) ;
#90014=CARTESIAN_POINT ( 'NONE',  ( 185.6927083336747160, 6.551208109652275624, -3.782341765624998686 ) ) ;
#90149=ORIENTED_EDGE ( 'NONE', *, *, #91538, .T. ) ;
#90167=CARTESIAN_POINT ( 'NONE',  ( 111.3003809011547105, 6.719038074301505681, -3.769326045731886232 ) ) ;
#90185=VERTEX_POINT ( 'NONE', #3962 ) ;
#90211=CARTESIAN_POINT ( 'NONE',  ( 186.0677083336747444, -4.367472073101514418, -7.564683531250002702 ) ) ;
#90237=EDGE_CURVE ( 'NONE', #129597, #116188, #36816, .T. ) ;
#90296=( BOUNDED_CURVE ( )  B_SPLINE_CURVE ( 2, ( #58553, #38933, #119381, #39577, #79484, #27777, #78847 ),
 .UNSPECIFIED., .F., .F. ) 
 B_SPLINE_CURVE_WITH_KNOTS ( ( 3, 2, 2, 3 ),
 ( 0.8571428571428578724, 0.8809523809523817084, 0.9047619047619054333, 0.9285714285714292693 ),
 .UNSPECIFIED. ) 
 CURVE ( )  GEOMETRIC_REPRESENTATION_ITEM ( )  RATIONAL_B_SPLINE_CURVE ( ( 0.9999999999999956701, 0.8660254037844430375, 1.000000000000000000, 0.8660254037844387076, 1.000000000000000000, 0.8660254037844349329, 1.000000000000003775 ) ) 
 REPRESENTATION_ITEM ( '' )  );
#90366=ORIENTED_EDGE ( 'NONE', *, *, #21071, .F. ) ;
#90448=ORIENTED_EDGE ( 'NONE', *, *, #64591, .F. ) ;
#90458=AXIS2_PLACEMENT_3D ( 'NONE', #86735, #97839, #8168 ) ;
#90462=CARTESIAN_POINT ( 'NONE',  ( 103.0345226653136450, 8.680034755040322736, 0.6735062902075328317 ) ) ;
#90469=EDGE_LOOP ( 'NONE', ( #82062, #32575, #90149, #34447, #32655 ) ) ;
#90516=DIRECTION ( 'NONE',  ( 0.000000000000000000, 0.000000000000000000, 1.000000000000000000 ) ) ;
#90550=CARTESIAN_POINT ( 'NONE',  ( 112.7289338494457809, 8.546997317143256723, 1.632411909918629167 ) ) ;
#90577=CARTESIAN_POINT ( 'NONE',  ( 186.0052083336747444, -6.551208109652278289, 3.782341765624995134 ) ) ;
#90625=ORIENTED_EDGE ( 'NONE', *, *, #1698, .F. ) ;
#90669=ADVANCED_FACE ( 'NONE', ( #51645 ), #3815, .F. ) ;
#90674=CARTESIAN_POINT ( 'NONE',  ( 184.1510416670080588, 4.367472073101518859, -7.564683531249999149 ) ) ;
#90725=FACE_OUTER_BOUND ( 'NONE', #98047, .T. ) ;
#90818=ORIENTED_EDGE ( 'NONE', *, *, #68426, .F. ) ;
#90849=DIRECTION ( 'NONE',  ( 0.000000000000000000, 0.000000000000000000, 1.000000000000000000 ) ) ;
#90874=CARTESIAN_POINT ( 'NONE',  ( 185.0260416670080588, -6.551208109652273848, -3.782341765625003571 ) ) ;
#90877=LINE ( 'NONE', #41162, #30391 ) ;
#90880=LINE ( 'NONE', #69290, #19798 ) ;
#90898=CARTESIAN_POINT ( 'NONE',  ( 186.1979166673494603, 6.668395609140176816, 3.850000000000000977 ) ) ;
#90954=EDGE_CURVE ( 'NONE', #121068, #15661, #50202, .T. ) ;
#90980=CARTESIAN_POINT ( 'NONE',  ( 184.6145833340161175, 6.668395609140177704, -3.849999999999998312 ) ) ;
#90997=AXIS2_PLACEMENT_3D ( 'NONE', #66836, #76027, #106764 ) ;
#91046=CARTESIAN_POINT ( 'NONE',  ( 186.3750000000000000, 8.891194145520236347, 5.444286225454521982E-16 ) ) ;
#91124=CARTESIAN_POINT ( 'NONE',  ( 184.6927083336747160, 6.551208109652275624, -3.782341765624998686 ) ) ;
#91153=CARTESIAN_POINT ( 'NONE',  ( 187.5000000000000000, 0.000000000000000000, 8.699999999999999289 ) ) ;
#91171=CARTESIAN_POINT ( 'NONE',  ( 187.2812500006828031, 0.000000000000000000, 7.700000000000000178 ) ) ;
#91336=ORIENTED_EDGE ( 'NONE', *, *, #100683, .F. ) ;
#91402=EDGE_CURVE ( 'NONE', #57508, #85963, #63567, .T. ) ;
#91406=CIRCLE ( 'NONE', #85141, 7.700000000000000178 ) ;
#91443=CARTESIAN_POINT ( 'NONE',  ( 129.5000000000000000, 0.6250000000000000000, 7.634788798650556707 ) ) ;
#91470=CARTESIAN_POINT ( 'NONE',  ( 187.1145833340161175, 6.668395609140177704, -3.849999999999998312 ) ) ;
#91524=CARTESIAN_POINT ( 'NONE',  ( 186.4218750003414016, 0.000000000000000000, 7.564683531250000925 ) ) ;
#91538=EDGE_CURVE ( 'NONE', #75118, #109041, #38350, .T. ) ;
#91648=CARTESIAN_POINT ( 'NONE',  ( 103.4640010755897919, 7.406936539094362892, 2.109949502027294255 ) ) ;
#91760=FACE_OUTER_BOUND ( 'NONE', #50740, .T. ) ;
#91764=CARTESIAN_POINT ( 'NONE',  ( 184.6093750003413732, 9.264065473108010111E-16, -7.564683531250000925 ) ) ;
#91765=CIRCLE ( 'NONE', #112617, 3.000000000000000444 ) ;
#91797=DIRECTION ( 'NONE',  ( 1.000000000000000000, 0.000000000000000000, 0.000000000000000000 ) ) ;
#91832=ADVANCED_FACE ( 'NONE', ( #100853 ), #121784, .F. ) ;
#91862=ORIENTED_EDGE ( 'NONE', *, *, #23975, .T. ) ;
#91929=CARTESIAN_POINT ( 'NONE',  ( 129.5000000000000000, 0.000000000000000000, 6.000000000000000000 ) ) ;
#91969=CARTESIAN_POINT ( 'NONE',  ( 179.5000000000000000, 0.000000000000000000, 0.000000000000000000 ) ) ;
#92050=PLANE ( 'NONE',  #61066 ) ;
#92063=CARTESIAN_POINT ( 'NONE',  ( 187.5000000000000000, 9.429780353434619030E-16, -7.700000000000000178 ) ) ;
#92119=CARTESIAN_POINT ( 'NONE',  ( 179.5000000000000000, -0.6250000000000003331, 6.000000000000000000 ) ) ;
#92123=FACE_OUTER_BOUND ( 'NONE', #71728, .T. ) ;
#92157=CARTESIAN_POINT ( 'NONE',  ( 186.7968750003414300, 8.734944146203032389, 5.348610694689227483E-16 ) ) ;
#92400=CARTESIAN_POINT ( 'NONE',  ( 185.4010416670080872, -4.367472073101520635, 7.564683531249999149 ) ) ;
#92441=ORIENTED_EDGE ( 'NONE', *, *, #81594, .T. ) ;
#92459=ORIENTED_EDGE ( 'NONE', *, *, #42622, .T. ) ;
#92513=CARTESIAN_POINT ( 'NONE',  ( 187.2083333333333428, -4.445597072760115509, -7.700000000000001954 ) ) ;
#92614=FACE_OUTER_BOUND ( 'NONE', #103629, .T. ) ;
#92623=CARTESIAN_POINT ( 'NONE',  ( 129.5000000000000000, 0.6250000000000000000, 7.634788798650556707 ) ) ;
#92687=FACE_OUTER_BOUND ( 'NONE', #101112, .T. ) ;
#92765=VERTEX_POINT ( 'NONE', #73033 ) ;
#92775=CARTESIAN_POINT ( 'NONE',  ( 186.1979166673494603, 6.668395609140176816, 3.850000000000000977 ) ) ;
#92781=EDGE_CURVE ( 'NONE', #57508, #93739, #12801, .T. ) ;
#92783=CARTESIAN_POINT ( 'NONE',  ( 187.5000000000000000, -1.500000000000000000, -6.000000000000000000 ) ) ;
#92793=DIRECTION ( 'NONE',  ( 1.000000000000000000, 0.000000000000000000, -0.000000000000000000 ) ) ;
#92823=CARTESIAN_POINT ( 'NONE',  ( 184.5677083336747444, -4.367472073101514418, -7.564683531250002702 ) ) ;
#92845=FACE_BOUND ( 'NONE', #11683, .T. ) ;
#92851=CARTESIAN_POINT ( 'NONE',  ( 185.2500000000000000, 9.429780353434619030E-16, -7.700000000000000178 ) ) ;
#92895=CARTESIAN_POINT ( 'NONE',  ( 186.5052083336747444, -6.551208109652278289, 3.782341765624995134 ) ) ;
#92896=CARTESIAN_POINT ( 'NONE',  ( 184.0000000000000000, 0.000000000000000000, 7.700000000000000178 ) ) ;
#93069=CARTESIAN_POINT ( 'NONE',  ( 185.5260416670080588, -6.551208109652273848, -3.782341765625003571 ) ) ;
#93099=CARTESIAN_POINT ( 'NONE',  ( 129.5000000000000000, 1.500000000000000000, -6.000000000000000000 ) ) ;
#93181=CARTESIAN_POINT ( 'NONE',  ( 187.0416666666666288, -4.445597072760122614, 7.699999999999998401 ) ) ;
#93229=ORIENTED_EDGE ( 'NONE', *, *, #3193, .T. ) ;
#93256=ORIENTED_EDGE ( 'NONE', *, *, #116510, .T. ) ;
#93278=DIRECTION ( 'NONE',  ( 0.000000000000000000, 0.000000000000000000, -1.000000000000000000 ) ) ;
#93410=CARTESIAN_POINT ( 'NONE',  ( 186.6979166673494603, 6.668395609140176816, 3.850000000000000977 ) ) ;
#93453=CARTESIAN_POINT ( 'NONE',  ( 186.0468750003414300, -8.734944146203032389, -1.604583208406768146E-15 ) ) ;
#93615=CARTESIAN_POINT ( 'NONE',  ( 185.7812500006828031, 0.000000000000000000, 7.700000000000000178 ) ) ;
#93667=CARTESIAN_POINT ( 'NONE',  ( 129.5000000000000000, 1.375000000000002442, -6.000000000000000888 ) ) ;
#93700=CARTESIAN_POINT ( 'NONE',  ( 184.3177083336747160, 4.367472073101515306, 7.564683531250000925 ) ) ;
#93739=VERTEX_POINT ( 'NONE', #24113 ) ;
#93772=FACE_OUTER_BOUND ( 'NONE', #65880, .T. ) ;
#93814=CARTESIAN_POINT ( 'NONE',  ( 185.6302083336747444, -4.367472073101514418, -7.564683531250002702 ) ) ;
#93977=CYLINDRICAL_SURFACE ( 'NONE', #17509, 8.699999999999999289 ) ;
#94055=CARTESIAN_POINT ( 'NONE',  ( 185.6979166673494603, 6.668395609140176816, 3.850000000000000977 ) ) ;
#94098=CARTESIAN_POINT ( 'NONE',  ( 184.2968750003414300, 8.734944146203032389, 5.348610694689227483E-16 ) ) ;
#94142=VERTEX_POINT ( 'NONE', #46828 ) ;
#94162=B_SPLINE_CURVE_WITH_KNOTS ( 'NONE', 3,
 ( #68253, #60401, #8670, #50542, #49937, #119288, #59096, #80672, #20459, #68900, #108175, #79383, #100309, #120586, #9989, #90462, #108815, #99015, #18515, #89830, #119946, #19135, #48628, #9343, #805, #88539, #28996, #38837, #49290, #89192, #30296, #40764, #30935, #57806, #97718, #53773 ),
 .UNSPECIFIED., .F., .F.,
 ( 4, 2, 2, 2, 2, 2, 2, 2, 2, 2, 2, 2, 2, 2, 2, 2, 2, 4 ),
 ( 0.01599712308563960503, 0.01699497736294824229, 0.01799283164025687956, 0.01899068591756551683, 0.01998854019487415062, 0.02098639447218278789, 0.02198424874949142516, 0.02298210302680006242, 0.02397995730410869969, 0.02447888444276301659, 0.02497781158141733349, 0.02597566585872598116, 0.02697352013603462537, 0.02797137441334326957, 0.02896922869065191725, 0.02996708296796055798, 0.03096493724526920219, 0.03196279152257784639 ),
 .UNSPECIFIED. ) ;
#94184=ADVANCED_FACE ( 'NONE', ( #57935 ), #46167, .F. ) ;
#94263=VERTEX_POINT ( 'NONE', #10728 ) ;
#94355=VERTEX_POINT ( 'NONE', #2879 ) ;
#94438=CARTESIAN_POINT ( 'NONE',  ( 184.3802083336747444, 4.367472073101515306, 7.564683531250000925 ) ) ;
#94610=VECTOR ( 'NONE', #39350, 1000.000000000000000 ) ;
#94616=DIRECTION ( 'NONE',  ( 0.000000000000000000, 0.000000000000000000, 1.000000000000000000 ) ) ;
#94670=CARTESIAN_POINT ( 'NONE',  ( 186.9166666666666856, 6.668395609140176816, 3.850000000000000977 ) ) ;
#94681=LINE ( 'NONE', #117517, #2865 ) ;
#94688=CARTESIAN_POINT ( 'NONE',  ( 184.9479166673494603, -6.668395609140176816, -3.850000000000003642 ) ) ;
#94734=CARTESIAN_POINT ( 'NONE',  ( 184.5052083336747444, -6.551208109652278289, 3.782341765624995134 ) ) ;
#94821=ORIENTED_EDGE ( 'NONE', *, *, #6678, .F. ) ;
#94900=DIRECTION ( 'NONE',  ( 0.000000000000000000, -1.000000000000000000, -0.000000000000000000 ) ) ;
#95004=DIRECTION ( 'NONE',  ( -1.000000000000000000, -0.000000000000000000, -0.000000000000000000 ) ) ;
#95049=DIRECTION ( 'NONE',  ( -1.000000000000000000, -0.000000000000000000, -0.000000000000000000 ) ) ;
#95062=CARTESIAN_POINT ( 'NONE',  ( 185.0312500006828031, 9.429780353434619030E-16, -7.700000000000000178 ) ) ;
#95088=EDGE_CURVE ( 'NONE', #62383, #43268, #106703, .T. ) ;
#95103=CARTESIAN_POINT ( 'NONE',  ( 184.0885416670080872, -6.551208109652273848, -3.782341765625003571 ) ) ;
#95127=DIRECTION ( 'NONE',  ( 0.000000000000000000, 0.000000000000000000, -1.000000000000000000 ) ) ;
#95235=ORIENTED_EDGE ( 'NONE', *, *, #38255, .T. ) ;
#95284=ORIENTED_EDGE ( 'NONE', *, *, #59684, .F. ) ;
#95299=CARTESIAN_POINT ( 'NONE',  ( 129.5000000000000000, -0.6250000000000000000, 7.634788798650553154 ) ) ;
#95325=CARTESIAN_POINT ( 'NONE',  ( 186.7500000000000000, 9.429780353434619030E-16, -7.700000000000000178 ) ) ;
#95338=EDGE_LOOP ( 'NONE', ( #73328, #59603, #68746, #108077, #6275, #79544, #68593, #112317, #5616, #23181, #97196, #17633, #27369, #17954, #34971, #66961, #15467 ) ) ;
#95346=CARTESIAN_POINT ( 'NONE',  ( 187.3177083336747444, 4.367472073101515306, 7.564683531250000925 ) ) ;
#95349=CARTESIAN_POINT ( 'NONE',  ( 179.5000000000000000, -0.6250000000000028866, -7.634788798650553154 ) ) ;
#95388=CARTESIAN_POINT ( 'NONE',  ( 184.7552083336747444, 6.551208109652275624, -3.782341765624998686 ) ) ;
#95562=ORIENTED_EDGE ( 'NONE', *, *, #82357, .F. ) ;
#95608=ORIENTED_EDGE ( 'NONE', *, *, #108357, .F. ) ;
#95703=ORIENTED_EDGE ( 'NONE', *, *, #60247, .T. ) ;
#95745=CARTESIAN_POINT ( 'NONE',  ( 186.6250000000000284, -8.891194145520236347, -1.633285867636356693E-15 ) ) ;
#95913=CARTESIAN_POINT ( 'NONE',  ( 179.5000000000000000, -0.6250000000000028866, -7.634788798650553154 ) ) ;
#95990=CARTESIAN_POINT ( 'NONE',  ( 186.7760416670080588, 6.551208109652274736, 3.782341765625001351 ) ) ;
#96001=LINE ( 'NONE', #25299, #63451 ) ;
#96080=ORIENTED_EDGE ( 'NONE', *, *, #112266, .F. ) ;
#96095=CARTESIAN_POINT ( 'NONE',  ( 184.8802083336747444, 4.367472073101515306, 7.564683531250000925 ) ) ;
#96236=DIRECTION ( 'NONE',  ( -1.000000000000000000, 0.000000000000000000, 0.000000000000000000 ) ) ;
#96248=DIRECTION ( 'NONE',  ( 0.000000000000000000, -1.846105847067148515E-16, -1.000000000000000000 ) ) ;
#96355=AXIS2_PLACEMENT_3D ( 'NONE', #6439, #127546, #97431 ) ;
#96365=CARTESIAN_POINT ( 'NONE',  ( 186.0833333333333144, -6.668395609140180369, 3.849999999999994760 ) ) ;
#96404=DIRECTION ( 'NONE',  ( 0.000000000000000000, 0.000000000000000000, 1.000000000000000000 ) ) ;
#96435=EDGE_CURVE ( 'NONE', #85963, #110378, #92, .T. ) ;
#96597=CARTESIAN_POINT ( 'NONE',  ( 129.5000000000000000, -1.375000000000000000, 7.634788798650553154 ) ) ;
#96607=CARTESIAN_POINT ( 'NONE',  ( 186.8177083336747160, 4.367472073101515306, 7.564683531250000925 ) ) ;
#96651=CARTESIAN_POINT ( 'NONE',  ( 185.5885416670080872, -6.551208109652273848, -3.782341765625003571 ) ) ;
#96726=CARTESIAN_POINT ( 'NONE',  ( 184.2968750003414300, 8.734944146203032389, 5.348610694689227483E-16 ) ) ;
#96753=VECTOR ( 'NONE', #106642, 1000.000000000000000 ) ;
#96767=DIRECTION ( 'NONE',  ( -1.000000000000000000, 0.000000000000000000, 0.000000000000000000 ) ) ;
#96784=AXIS2_PLACEMENT_3D ( 'NONE', #74497, #114411, #24756 ) ;
#96801=CARTESIAN_POINT ( 'NONE',  ( 187.0416666666666572, -4.445597072760107515, 7.700000000000023270 ) ) ;
#96973=EDGE_CURVE ( 'NONE', #65955, #4435, #88899, .T. ) ;
#97029=CARTESIAN_POINT ( 'NONE',  ( 186.1666666666666856, -6.668395609140176816, -3.850000000000003642 ) ) ;
#97063=CARTESIAN_POINT ( 'NONE',  ( 129.5000000000000000, 0.6250000000000000000, 7.634788798650556707 ) ) ;
#97181=VECTOR ( 'NONE', #88204, 1000.000000000000000 ) ;
#97196=ORIENTED_EDGE ( 'NONE', *, *, #91402, .T. ) ;
#97228=ORIENTED_EDGE ( 'NONE', *, *, #86187, .T. ) ;
#97272=CARTESIAN_POINT ( 'NONE',  ( 183.9895833340161175, -4.445597072760115509, -7.700000000000001954 ) ) ;
#97274=CARTESIAN_POINT ( 'NONE',  ( 129.5000000000000000, -0.6250000000000024425, -6.000000000000000000 ) ) ;
#97383=CARTESIAN_POINT ( 'NONE',  ( 186.1718750003414016, 9.264065473108010111E-16, -7.564683531250000925 ) ) ;
#97399=LINE ( 'NONE', #126220, #10128 ) ;
#97408=CARTESIAN_POINT ( 'NONE',  ( 187.5000000000000000, 0.000000000000000000, 0.000000000000000000 ) ) ;
#97429=CARTESIAN_POINT ( 'NONE',  ( 112.4769073329632931, 7.370384220483499504, 2.250641841625343531 ) ) ;
#97431=DIRECTION ( 'NONE',  ( 0.000000000000000000, 0.000000000000000000, -1.000000000000000000 ) ) ;
#97447=VERTEX_POINT ( 'NONE', #62524 ) ;
#97449=ORIENTED_EDGE ( 'NONE', *, *, #24597, .F. ) ;
#97562=LINE ( 'NONE', #48467, #47257 ) ;
#97591=CARTESIAN_POINT ( 'NONE',  ( 187.5000000000000000, 0.000000000000000000, 7.700000000000000178 ) ) ;
#97624=CIRCLE ( 'NONE', #16116, 7.700000000000000178 ) ;
#97671=CARTESIAN_POINT ( 'NONE',  ( 185.6250000000000284, -8.891194145520236347, -1.633285867636356693E-15 ) ) ;
#97705=EDGE_CURVE ( 'NONE', #80059, #2046, #30170, .T. ) ;
#97718=CARTESIAN_POINT ( 'NONE',  ( 107.6617659101945748, 7.119691004531019551, -5.000000000000002665 ) ) ;
#97746=VECTOR ( 'NONE', #109999, 1000.000000000000000 ) ;
#97769=EDGE_CURVE ( 'NONE', #41599, #51279, #124181, .T. ) ;
#97787=CARTESIAN_POINT ( 'NONE',  ( 179.5000000000000000, 1.375000000000002442, -7.576237522675751457 ) ) ;
#97795=CARTESIAN_POINT ( 'NONE',  ( 111.0583702135628528, 7.744754444937881566, -3.968742208708922359 ) ) ;
#97839=DIRECTION ( 'NONE',  ( -1.000000000000000000, -0.000000000000000000, -0.000000000000000000 ) ) ;
#97903=EDGE_CURVE ( 'NONE', #113580, #114828, #15645, .T. ) ;
#97911=CARTESIAN_POINT ( 'NONE',  ( 185.0677083336747160, -4.367472073101514418, -7.564683531250002702 ) ) ;
#97933=LINE ( 'NONE', #61898, #55988 ) ;
#98027=CARTESIAN_POINT ( 'NONE',  ( 185.9635416670080588, -4.367472073101520635, 7.564683531249999149 ) ) ;
#98047=EDGE_LOOP ( 'NONE', ( #69318, #63478, #40696, #74252, #105983, #1966, #91336, #63016, #90366, #13720, #57437, #67202, #15731, #65058 ) ) ;
#98075=CARTESIAN_POINT ( 'NONE',  ( 112.9334202320777365, 7.656891339828185039, 0.8302582904282872489 ) ) ;
#98102=DIRECTION ( 'NONE',  ( 0.000000000000000000, 0.000000000000000000, -1.000000000000000000 ) ) ;
#98110=CARTESIAN_POINT ( 'NONE',  ( 186.2760416670080588, 6.551208109652274736, 3.782341765625001351 ) ) ;
#98128=ADVANCED_FACE ( 'NONE', ( #50942 ), #81042, .T. ) ;
#98181=CARTESIAN_POINT ( 'NONE',  ( 187.5000000000000000, -1.500000000000000000, -6.000000000000000000 ) ) ;
#98200=DIRECTION ( 'NONE',  ( 0.000000000000000000, 0.000000000000000000, 1.000000000000000000 ) ) ;
#98204=FACE_OUTER_BOUND ( 'NONE', #73643, .T. ) ;
#98305=CARTESIAN_POINT ( 'NONE',  ( 185.6666666666666856, -6.668395609140176816, -3.850000000000003642 ) ) ;
#98340=CARTESIAN_POINT ( 'NONE',  ( 187.5000000000000000, 9.429780353434619030E-16, -7.700000000000000178 ) ) ;
#98349=CARTESIAN_POINT ( 'NONE',  ( 186.4427083336747160, -6.551208109652278289, 3.782341765624995134 ) ) ;
#98414=DIRECTION ( 'NONE',  ( 0.000000000000000000, 0.000000000000000000, 1.000000000000000000 ) ) ;
#98423=CARTESIAN_POINT ( 'NONE',  ( 108.3381794683780583, 7.119691004531020440, 5.000000000000002665 ) ) ;
#98510=EDGE_LOOP ( 'NONE', ( #10538, #20903, #81722, #97449, #12682 ) ) ;
#98540=CARTESIAN_POINT ( 'NONE',  ( 186.0260416670080588, -6.551208109652273848, -3.782341765625003571 ) ) ;
#98544=ORIENTED_EDGE ( 'NONE', *, *, #14729, .T. ) ;
#98558=ORIENTED_EDGE ( 'NONE', *, *, #31260, .F. ) ;
#98605=AXIS2_PLACEMENT_3D ( 'NONE', #33706, #44167, #85384 ) ;
#98660=CARTESIAN_POINT ( 'NONE',  ( 186.4218750003414016, 0.000000000000000000, 7.564683531250000925 ) ) ;
#98707=CARTESIAN_POINT ( 'NONE',  ( 112.9640574409401808, 7.676535526101522677, -0.6848668807478225373 ) ) ;
#98743=CARTESIAN_POINT ( 'NONE',  ( 179.5000000000000000, -0.6250000000000003331, 6.000000000000000000 ) ) ;
#98749=CARTESIAN_POINT ( 'NONE',  ( 185.6927083336747160, 6.551208109652275624, -3.782341765624998686 ) ) ;
#98769=AXIS2_PLACEMENT_3D ( 'NONE', #29362, #39832, #128200 ) ;
#98836=EDGE_LOOP ( 'NONE', ( #93229, #42940 ) ) ;
#98869=CARTESIAN_POINT ( 'NONE',  ( 179.5000000000000000, -0.6250000000000000000, 7.634788798650553154 ) ) ;
#98896=FILL_AREA_STYLE_COLOUR ( '', #116695 ) ;
#99001=DIRECTION ( 'NONE',  ( 0.000000000000000000, 0.000000000000000000, 1.000000000000000000 ) ) ;
#99010=CARTESIAN_POINT ( 'NONE',  ( 186.8177083336747160, 4.367472073101515306, 7.564683531250000925 ) ) ;
#99015=CARTESIAN_POINT ( 'NONE',  ( 102.9998079663853900, 8.700110364096246940, -0.1627839287194029205 ) ) ;
#99099=CARTESIAN_POINT ( 'NONE',  ( 112.9585346383515230, 8.676224923738738326, 0.6641129214945534764 ) ) ;
#99125=CARTESIAN_POINT ( 'NONE',  ( 187.5000000000000000, -1.000000000000025535, -7.634788798650553154 ) ) ;
#99145=VERTEX_POINT ( 'NONE', #115302 ) ;
#99152=ORIENTED_EDGE ( 'NONE', *, *, #125351, .T. ) ;
#99174=EDGE_CURVE ( 'NONE', #69479, #85617, #66228, .T. ) ;
#99219=CARTESIAN_POINT ( 'NONE',  ( 184.0260416670080588, -6.551208109652273848, -3.782341765625003571 ) ) ;
#99354=CARTESIAN_POINT ( 'NONE',  ( 187.5000000000000000, 1.500000000000000000, 6.000000000000000000 ) ) ;
#99381=DIRECTION ( 'NONE',  ( 1.000000000000000000, 0.000000000000000000, 0.000000000000000000 ) ) ;
#99390=ORIENTED_EDGE ( 'NONE', *, *, #99174, .T. ) ;
#99426=CARTESIAN_POINT ( 'NONE',  ( 185.4427083336747160, -6.551208109652278289, 3.782341765624995134 ) ) ;
#99521=EDGE_CURVE ( 'NONE', #84030, #74365, #5054, .T. ) ;
#99551=CARTESIAN_POINT ( 'NONE',  ( 105.4725005298439271, 6.373511028144405621, 4.325813758252836649 ) ) ;
#99559=LINE ( 'NONE', #48514, #18425 ) ;
#99589=CYLINDRICAL_SURFACE ( 'NONE', #117324, 8.699999999999999289 ) ;
#99658=EDGE_CURVE ( 'NONE', #1000, #83312, #87477, .T. ) ;
#99745=CARTESIAN_POINT ( 'NONE',  ( 112.8268375934096071, 8.601552705179036806, 1.314999179819271946 ) ) ;
#99768=EDGE_CURVE ( 'NONE', #23165, #55407, #24801, .T. ) ;
#99769=CARTESIAN_POINT ( 'NONE',  ( 186.9635416670080303, -4.367472073101519747, 7.564683531249999149 ) ) ;
#99782=AXIS2_PLACEMENT_3D ( 'NONE', #32680, #66610, #37174 ) ;
#99802=VERTEX_POINT ( 'NONE', #62724 ) ;
#99864=CARTESIAN_POINT ( 'NONE',  ( 185.5677083336747160, -4.367472073101514418, -7.564683531250002702 ) ) ;
#99939=ORIENTED_EDGE ( 'NONE', *, *, #83551, .T. ) ;
#99947=CARTESIAN_POINT ( 'NONE',  ( 127.5000000000000000, -1.500000000000000000, -6.000000000000000000 ) ) ;
#99948=ORIENTED_EDGE ( 'NONE', *, *, #68617, .T. ) ;
#99993=MECHANICAL_DESIGN_GEOMETRIC_PRESENTATION_REPRESENTATION('',(#28984),#81215);
#100021=CARTESIAN_POINT ( 'NONE',  ( 110.5285083638605244, 6.373905227100763682, 4.325246220449017187 ) ) ;
#100058=CARTESIAN_POINT ( 'NONE',  ( 185.3177083336747160, 4.367472073101515306, 7.564683531250000925 ) ) ;
#100071=ORIENTED_EDGE ( 'NONE', *, *, #81186, .F. ) ;
#100075=ORIENTED_EDGE ( 'NONE', *, *, #10204, .F. ) ;
#100114=CARTESIAN_POINT ( 'NONE',  ( 187.2916666666666572, 4.445597072760113733, -7.700000000000009948 ) ) ;
#100140=CARTESIAN_POINT ( 'NONE',  ( 187.5000000000000000, -1.500000000000000000, -6.000000000000000000 ) ) ;
#100155=CARTESIAN_POINT ( 'NONE',  ( 179.5000000000000000, 0.000000000000000000, -6.000000000000000000 ) ) ;
#100289=ADVANCED_FACE ( 'NONE', ( #90725 ), #109727, .F. ) ;
#100307=CARTESIAN_POINT ( 'NONE',  ( 186.4843750003414016, -8.734944146203032389, -1.604583208406767949E-15 ) ) ;
#100309=CARTESIAN_POINT ( 'NONE',  ( 103.5210970489751361, 8.410658075108495169, 2.246395211621319277 ) ) ;
#100365=ORIENTED_EDGE ( 'NONE', *, *, #16541, .F. ) ;
#100411=CARTESIAN_POINT ( 'NONE',  ( 186.1302083336747444, -4.367472073101514418, -7.564683531250002702 ) ) ;
#100491=CARTESIAN_POINT ( 'NONE',  ( 184.1093750003413732, 9.264065473108010111E-16, -7.564683531250000925 ) ) ;
#100576=FACE_OUTER_BOUND ( 'NONE', #56032, .T. ) ;
#100578=AXIS2_PLACEMENT_3D ( 'NONE', #27471, #67375, #5260 ) ;
#100607=LINE ( 'NONE', #102545, #106671 ) ;
#100680=CARTESIAN_POINT ( 'NONE',  ( 185.3593750003413732, 0.000000000000000000, 7.564683531250000925 ) ) ;
#100683=EDGE_CURVE ( 'NONE', #114828, #26322, #37466, .T. ) ;
#100704=DIRECTION ( 'NONE',  ( 0.000000000000000000, 0.000000000000000000, 1.000000000000000000 ) ) ;
#100708=CARTESIAN_POINT ( 'NONE',  ( 186.0312500006828031, 9.429780353434619030E-16, -7.700000000000000178 ) ) ;
#100714=VERTEX_POINT ( 'NONE', #104882 ) ;
#100740=LINE ( 'NONE', #18319, #7411 ) ;
#100805=CARTESIAN_POINT ( 'NONE',  ( 103.5362392592695642, 7.362830575048670667, 2.258572230843124196 ) ) ;
#100853=FACE_OUTER_BOUND ( 'NONE', #603, .T. ) ;
#100883=CARTESIAN_POINT ( 'NONE',  ( 184.0416666666666572, -4.445597072760122614, 7.699999999999998401 ) ) ;
#100895=ORIENTED_EDGE ( 'NONE', *, *, #10269, .T. ) ;
#100928=CARTESIAN_POINT ( 'NONE',  ( 186.2760416670080588, 6.551208109652274736, 3.782341765625001351 ) ) ;
#100939=ORIENTED_EDGE ( 'NONE', *, *, #25318, .T. ) ;
#100984=CARTESIAN_POINT ( 'NONE',  ( 185.0416666666667140, -4.445597072760063107, 7.700000000000102318 ) ) ;
#101013=LINE ( 'NONE', #41478, #80550 ) ;
#101049=CARTESIAN_POINT ( 'NONE',  ( 186.5468750003414300, -8.734944146203032389, -1.604583208406768146E-15 ) ) ;
#101070=VECTOR ( 'NONE', #46909, 1000.000000000000000 ) ;
#101112=EDGE_LOOP ( 'NONE', ( #64152, #67688, #40333, #106411 ) ) ;
#101185=EDGE_CURVE ( 'NONE', #63648, #111056, #116319, .T. ) ;
#101214=ORIENTED_EDGE ( 'NONE', *, *, #89301, .T. ) ;
#101288=VECTOR ( 'NONE', #83357, 1000.000000000000000 ) ;
#101305=CARTESIAN_POINT ( 'NONE',  ( 186.6145833340161175, 6.668395609140177704, -3.849999999999998312 ) ) ;
#101351=CARTESIAN_POINT ( 'NONE',  ( 186.8385416670080872, 6.551208109652274736, 3.782341765625001351 ) ) ;
#101416=CARTESIAN_POINT ( 'NONE',  ( 184.1249999999999716, -8.891194145520236347, -1.633285867636356299E-15 ) ) ;
#101545=CARTESIAN_POINT ( 'NONE',  ( 184.1250000000000284, -8.891194145520236347, -1.633285867636356693E-15 ) ) ;
#101564=VERTEX_POINT ( 'NONE', #117435 ) ;
#101570=AXIS2_PLACEMENT_3D ( 'NONE', #39570, #20548, #21849 ) ;
#101592=CARTESIAN_POINT ( 'NONE',  ( 184.6510416670080588, 4.367472073101518859, -7.564683531249999149 ) ) ;
#101636=ORIENTED_EDGE ( 'NONE', *, *, #11245, .T. ) ;
#101657=CARTESIAN_POINT ( 'NONE',  ( 185.2395833340161460, 4.445597072760175905, 7.699999999999896261 ) ) ;
#101699=DIRECTION ( 'NONE',  ( 0.000000000000000000, 0.000000000000000000, -1.000000000000000000 ) ) ;
#101712=CARTESIAN_POINT ( 'NONE',  ( 184.3750000000000000, 8.891194145520236347, 5.444286225454521982E-16 ) ) ;
#101765=ORIENTED_EDGE ( 'NONE', *, *, #12913, .F. ) ;
#101784=ORIENTED_EDGE ( 'NONE', *, *, #118755, .F. ) ;
#101808=LINE ( 'NONE', #92623, #61503 ) ;
#101822=FACE_OUTER_BOUND ( 'NONE', #52111, .T. ) ;
#101836=DIRECTION ( 'NONE',  ( 0.000000000000000000, 0.000000000000000000, 1.000000000000000000 ) ) ;
#101993=CARTESIAN_POINT ( 'NONE',  ( 184.6093750003413732, 9.264065473108010111E-16, -7.564683531250000925 ) ) ;
#102062=CARTESIAN_POINT ( 'NONE',  ( 184.0833333333333144, -6.668395609140180369, 3.849999999999994760 ) ) ;
#102067=VERTEX_POINT ( 'NONE', #28952 ) ;
#102100=ORIENTED_EDGE ( 'NONE', *, *, #55526, .T. ) ;
#102120=CARTESIAN_POINT ( 'NONE',  ( 107.3227259355851402, 5.885842102929867536, -4.965337704341070690 ) ) ;
#102236=PLANE ( 'NONE',  #110374 ) ;
#102239=CARTESIAN_POINT ( 'NONE',  ( 183.9843750003414016, -8.734944146203032389, -1.604583208406767949E-15 ) ) ;
#102240=VECTOR ( 'NONE', #33774, 1000.000000000000000 ) ;
#102415=CARTESIAN_POINT ( 'NONE',  ( 129.5000000000000000, 0.9999999999999985567, 7.634788798650556707 ) ) ;
#102518=CARTESIAN_POINT ( 'NONE',  ( 129.5000000000000000, 1.500000000000000000, 0.000000000000000000 ) ) ;
#102545=CARTESIAN_POINT ( 'NONE',  ( 179.5000000000000000, 1.375000000000000000, 7.634788798650556707 ) ) ;
#102571=CARTESIAN_POINT ( 'NONE',  ( 187.0729166673494319, 4.445597072760120838, -7.699999999999998401 ) ) ;
#102618=CARTESIAN_POINT ( 'NONE',  ( 184.4427083336747160, -6.551208109652278289, 3.782341765624995134 ) ) ;
#102632=AXIS2_PLACEMENT_3D ( 'NONE', #2305, #13422, #83481 ) ;
#102652=DIRECTION ( 'NONE',  ( -1.000000000000000000, -0.000000000000000000, -0.000000000000000000 ) ) ;
#102711=ORIENTED_EDGE ( 'NONE', *, *, #24430, .F. ) ;
#102743=CARTESIAN_POINT ( 'NONE',  ( 103.5236730166301697, 7.370027598015842507, -2.251927279840987506 ) ) ;
#102860=VECTOR ( 'NONE', #118515, 1000.000000000000000 ) ;
#102886=CARTESIAN_POINT ( 'NONE',  ( 184.4895833340161460, -4.445597072760175017, -7.699999999999898037 ) ) ;
#102970=DIRECTION ( 'NONE',  ( 0.000000000000000000, -0.000000000000000000, -1.000000000000000000 ) ) ;
#102977=CARTESIAN_POINT ( 'NONE',  ( 185.2968750003414300, 8.734944146203032389, 5.348610694689227483E-16 ) ) ;
#103003=ADVANCED_FACE ( 'NONE', ( #64994 ), #33629, .T. ) ;
#103025=DIRECTION ( 'NONE',  ( -1.000000000000000000, -0.000000000000000000, -0.000000000000000000 ) ) ;
#103093=PLANE ( 'NONE',  #24871 ) ;
#103169=FACE_OUTER_BOUND ( 'NONE', #128796, .T. ) ;
#103176=VERTEX_POINT ( 'NONE', #32136 ) ;
#103213=DIRECTION ( 'NONE',  ( 1.000000000000000000, 0.000000000000000000, 0.000000000000000000 ) ) ;
#103234=CARTESIAN_POINT ( 'NONE',  ( 186.5312500006828031, 9.429780353434619030E-16, -7.700000000000000178 ) ) ;
#103283=CARTESIAN_POINT ( 'NONE',  ( 184.8177083336747160, 4.367472073101515306, 7.564683531250000925 ) ) ;
#103409=CARTESIAN_POINT ( 'NONE',  ( 104.2471014634786712, 6.952484616901103642, -3.319144779746969309 ) ) ;
#103442=CARTESIAN_POINT ( 'NONE',  ( 185.8645833340161175, -6.668395609140180369, 3.849999999999994760 ) ) ;
#103447=DIRECTION ( 'NONE',  ( -1.000000000000000000, -0.000000000000000000, -0.000000000000000000 ) ) ;
#103515=ORIENTED_EDGE ( 'NONE', *, *, #99521, .F. ) ;
#103525=CARTESIAN_POINT ( 'NONE',  ( 184.9010416670080588, -4.367472073101520635, 7.564683531249999149 ) ) ;
#103629=EDGE_LOOP ( 'NONE', ( #103515, #37245, #95608, #21537, #73438 ) ) ;
#103637=CARTESIAN_POINT ( 'NONE',  ( 184.5468750003414300, -8.734944146203032389, -1.604583208406768146E-15 ) ) ;
#103671=CARTESIAN_POINT ( 'NONE',  ( 186.7083333333333428, -4.445597072760135937, -7.699999999999966427 ) ) ;
#103713=( BOUNDED_CURVE ( )  B_SPLINE_CURVE ( 2, ( #52142, #81590, #112987, #31223, #42321, #41692, #33155 ),
 .UNSPECIFIED., .F., .F. ) 
 B_SPLINE_CURVE_WITH_KNOTS ( ( 3, 2, 2, 3 ),
 ( 0.2142857142857144681, 0.2380952380952383041, 0.2619047619047621955, 0.2857142857142859760 ),
 .UNSPECIFIED. ) 
 CURVE ( )  GEOMETRIC_REPRESENTATION_ITEM ( )  RATIONAL_B_SPLINE_CURVE ( ( 0.9999999999999988898, 0.8660254037844397068, 1.000000000000000000, 0.8660254037844387076, 1.000000000000000000, 0.8660254037844371533, 1.000000000000001554 ) ) 
 REPRESENTATION_ITEM ( '' )  );
#103839=FACE_OUTER_BOUND ( 'NONE', #12857, .T. ) ;
#103877=CARTESIAN_POINT ( 'NONE',  ( 185.6145833340161175, 6.668395609140177704, -3.849999999999998312 ) ) ;
#103921=CARTESIAN_POINT ( 'NONE',  ( 186.8802083336747444, 4.367472073101515306, 7.564683531250000925 ) ) ;
#103980=AXIS2_PLACEMENT_3D ( 'NONE', #34267, #65634, #25711 ) ;
#103993=CARTESIAN_POINT ( 'NONE',  ( 187.0885416670080872, -6.551208109652273848, -3.782341765625003571 ) ) ;
#104021=CARTESIAN_POINT ( 'NONE',  ( 179.5000000000000000, 0.6250000000000003331, 6.000000000000000000 ) ) ;
#104170=CARTESIAN_POINT ( 'NONE',  ( 108.0000000000000142, 7.119691004531021328, -5.000000000000004441 ) ) ;
#104230=SURFACE_STYLE_USAGE ( .BOTH. , #42765 ) ;
#104274=CARTESIAN_POINT ( 'NONE',  ( 184.4635416670080588, -4.367472073101519747, 7.564683531249999149 ) ) ;
#104275=CARTESIAN_POINT ( 'NONE',  ( 187.5000000000000000, 0.000000000000000000, 7.700000000000000178 ) ) ;
#104286=CARTESIAN_POINT ( 'NONE',  ( 88.00000000000001421, 0.000000000000000000, 0.000000000000000000 ) ) ;
#104322=FACE_OUTER_BOUND ( 'NONE', #114932, .T. ) ;
#104375=CARTESIAN_POINT ( 'NONE',  ( 184.6250000000000000, -8.891194145520236347, -1.633285867636356299E-15 ) ) ;
#104391=ADVANCED_FACE ( 'NONE', ( #45053 ), #124248, .F. ) ;
#104445=FACE_OUTER_BOUND ( 'NONE', #98510, .T. ) ;
#104460=( BOUNDED_CURVE ( )  B_SPLINE_CURVE ( 2, ( #53433, #89648, #19614, #29440, #23301, #100114, #83536 ),
 .UNSPECIFIED., .F., .F. ) 
 B_SPLINE_CURVE_WITH_KNOTS ( ( 3, 2, 2, 3 ),
 ( 0.000000000000000000, 0.02380952380952383249, 0.04761904761904766498, 0.07142857142857149400 ),
 .UNSPECIFIED. ) 
 CURVE ( )  GEOMETRIC_REPRESENTATION_ITEM ( )  RATIONAL_B_SPLINE_CURVE ( ( 1.000000000000000000, 0.8660254037844387076, 1.000000000000000000, 0.8660254037844387076, 1.000000000000000000, 0.8660254037844383745, 1.000000000000000444 ) ) 
 REPRESENTATION_ITEM ( '' )  );
#104482=VECTOR ( 'NONE', #4038, 1000.000000000000114 ) ;
#104510=CARTESIAN_POINT ( 'NONE',  ( 185.1979166673494603, 6.668395609140176816, 3.850000000000000977 ) ) ;
#104620=CARTESIAN_POINT ( 'NONE',  ( 186.6302083336747728, -4.367472073101514418, -7.564683531250002702 ) ) ;
#104650=CARTESIAN_POINT ( 'NONE',  ( 187.0312500006828031, 9.429780353434619030E-16, -7.700000000000000178 ) ) ;
#104805=DIRECTION ( 'NONE',  ( 1.000000000000000000, 0.000000000000000000, 0.000000000000000000 ) ) ;
#104820=ORIENTED_EDGE ( 'NONE', *, *, #13713, .F. ) ;
#104875=VECTOR ( 'NONE', #85826, 1000.000000000000000 ) ;
#104882=CARTESIAN_POINT ( 'NONE',  ( 186.0000000000000000, 0.000000000000000000, 7.700000000000000178 ) ) ;
#104898=CARTESIAN_POINT ( 'NONE',  ( 184.7135416670080872, 4.367472073101518859, -7.564683531249999149 ) ) ;
#104905=DIRECTION ( 'NONE',  ( 0.000000000000000000, 0.000000000000000000, -1.000000000000000000 ) ) ;
#104968=EDGE_CURVE ( 'NONE', #122603, #33034, #27809, .T. ) ;
#105021=CARTESIAN_POINT ( 'NONE',  ( 186.0416666666666572, -4.445597072760079982, 7.700000000000070344 ) ) ;
#105061=CARTESIAN_POINT ( 'NONE',  ( 186.5312500006828031, 9.429780353434619030E-16, -7.700000000000000178 ) ) ;
#105074=DIRECTION ( 'NONE',  ( -1.000000000000000000, 0.000000000000000000, 0.000000000000000000 ) ) ;
#105114=CARTESIAN_POINT ( 'NONE',  ( 127.5000000000000000, 0.000000000000000000, 0.000000000000000000 ) ) ;
#105149=CARTESIAN_POINT ( 'NONE',  ( 187.1093750003414016, 9.264065473108010111E-16, -7.564683531250000925 ) ) ;
#105399=VECTOR ( 'NONE', #78202, 1000.000000000000000 ) ;
#105565=CARTESIAN_POINT ( 'NONE',  ( 187.3333333333333144, 6.668395609140177704, -3.849999999999998312 ) ) ;
#105626=ORIENTED_EDGE ( 'NONE', *, *, #123720, .T. ) ;
#105650=ORIENTED_EDGE ( 'NONE', *, *, #49030, .F. ) ;
#105663=CARTESIAN_POINT ( 'NONE',  ( 184.0312500006828031, 9.429780353434619030E-16, -7.700000000000000178 ) ) ;
#105740=PLANE ( 'NONE',  #8735 ) ;
#105769=DIRECTION ( 'NONE',  ( 0.000000000000000000, 1.846105847067148761E-16, 1.000000000000000000 ) ) ;
#105809=CARTESIAN_POINT ( 'NONE',  ( 186.6927083336747160, 6.551208109652275624, -3.782341765624998686 ) ) ;
#105851=CARTESIAN_POINT ( 'NONE',  ( 185.0052083336747444, -6.551208109652278289, 3.782341765624995134 ) ) ;
#105924=CARTESIAN_POINT ( 'NONE',  ( 185.0885416670080872, -6.551208109652273848, -3.782341765625003571 ) ) ;
#105983=ORIENTED_EDGE ( 'NONE', *, *, #4467, .T. ) ;
#106088=CARTESIAN_POINT ( 'NONE',  ( 179.5000000000000000, -0.6250000000000000000, 7.634788798650553154 ) ) ;
#106150=ORIENTED_EDGE ( 'NONE', *, *, #126217, .T. ) ;
#106167=VECTOR ( 'NONE', #123670, 1000.000000000000114 ) ;
#106211=CARTESIAN_POINT ( 'NONE',  ( 185.4583333333333144, 4.445597072760117285, 7.699999999999999289 ) ) ;
#106240=ORIENTED_EDGE ( 'NONE', *, *, #108357, .T. ) ;
#106386=ORIENTED_EDGE ( 'NONE', *, *, #40576, .F. ) ;
#106411=ORIENTED_EDGE ( 'NONE', *, *, #12913, .T. ) ;
#106419=ORIENTED_EDGE ( 'NONE', *, *, #16541, .T. ) ;
#106447=CARTESIAN_POINT ( 'NONE',  ( 184.3229166673494603, -4.445597072760122614, 7.699999999999998401 ) ) ;
#106456=ORIENTED_EDGE ( 'NONE', *, *, #40576, .T. ) ;
#106522=ORIENTED_EDGE ( 'NONE', *, *, #51756, .T. ) ;
#106549=CARTESIAN_POINT ( 'NONE',  ( 127.5000000000000000, 1.500000000000000000, 6.000000000000000000 ) ) ;
#106553=CARTESIAN_POINT ( 'NONE',  ( 185.7552083336747444, 6.551208109652275624, -3.782341765624998686 ) ) ;
#106605=LINE ( 'NONE', #66040, #54937 ) ;
#106642=DIRECTION ( 'NONE',  ( 0.000000000000000000, -1.000000000000000000, -0.000000000000000000 ) ) ;
#106671=VECTOR ( 'NONE', #73097, 1000.000000000000000 ) ;
#106703=LINE ( 'NONE', #47160, #61526 ) ;
#106732=CARTESIAN_POINT ( 'NONE',  ( 185.6562500006828031, 8.891194145520236347, 5.444286225454521982E-16 ) ) ;
#106734=EDGE_CURVE ( 'NONE', #126401, #75118, #76789, .T. ) ;
#106764=DIRECTION ( 'NONE',  ( 0.000000000000000000, 1.846105847067148761E-16, 1.000000000000000000 ) ) ;
#106782=ADVANCED_FACE ( 'NONE', ( #57797 ), #48616, .F. ) ;
#106820=ORIENTED_EDGE ( 'NONE', *, *, #80456, .F. ) ;
#106831=CARTESIAN_POINT ( 'NONE',  ( 186.8333333333333144, 6.668395609140177704, -3.849999999999998312 ) ) ;
#106962=CARTESIAN_POINT ( 'NONE',  ( 183.9609375001707008, 0.000000000000000000, 7.632341765625000107 ) ) ;
#107078=CARTESIAN_POINT ( 'NONE',  ( 184.4062500006828316, -8.891194145520236347, -1.633285867636356693E-15 ) ) ;
#107090=CARTESIAN_POINT ( 'NONE',  ( 129.5000000000000000, 1.375000000000000222, 6.000000000000000000 ) ) ;
#107101=ORIENTED_EDGE ( 'NONE', *, *, #97769, .F. ) ;
#107122=CARTESIAN_POINT ( 'NONE',  ( 185.1718750003414016, 9.264065473108010111E-16, -7.564683531250000925 ) ) ;
#107151=CARTESIAN_POINT ( 'NONE',  ( 185.4166666666666856, 6.668395609140176816, 3.850000000000000977 ) ) ;
#107199=CARTESIAN_POINT ( 'NONE',  ( 184.4635416670080588, -4.367472073101520635, 7.564683531249999149 ) ) ;
#107251=CARTESIAN_POINT ( 'NONE',  ( 129.5000000000000000, 0.000000000000000000, 0.000000000000000000 ) ) ;
#107258=CARTESIAN_POINT ( 'NONE',  ( 179.5000000000000000, -1.375000000000002442, -6.000000000000000000 ) ) ;
#107287=ORIENTED_EDGE ( 'NONE', *, *, #24430, .T. ) ;
#107349=DIRECTION ( 'NONE',  ( 0.000000000000000000, 0.000000000000000000, -1.000000000000000000 ) ) ;
#107480=LINE ( 'NONE', #117932, #112135 ) ;
#107496=AXIS2_PLACEMENT_3D ( 'NONE', #98181, #49107, #68076 ) ;
#107498=CARTESIAN_POINT ( 'NONE',  ( 185.5833333333333144, -6.668395609140180369, 3.849999999999994760 ) ) ;
#107506=ORIENTED_EDGE ( 'NONE', *, *, #8037, .T. ) ;
#107545=VECTOR ( 'NONE', #55601, 1000.000000000000000 ) ;
#107624=LINE ( 'NONE', #106962, #52204 ) ;
#107701=CARTESIAN_POINT ( 'NONE',  ( 185.0000000000000000, 0.000000000000000000, 7.700000000000000178 ) ) ;
#107850=CARTESIAN_POINT ( 'NONE',  ( 184.0052083336747160, -6.551208109652278289, 3.782341765624995134 ) ) ;
#107865=VECTOR ( 'NONE', #16286, 1000.000000000000000 ) ;
#107895=CARTESIAN_POINT ( 'NONE',  ( 112.3213495094165921, 7.276123333567264595, 2.535987402356341125 ) ) ;
#107934=CARTESIAN_POINT ( 'NONE',  ( 186.3177083336747160, 4.367472073101515306, 7.564683531250000925 ) ) ;
#107967=AXIS2_PLACEMENT_3D ( 'NONE', #50287, #129520, #30012 ) ;
#107978=ORIENTED_EDGE ( 'NONE', *, *, #115420, .T. ) ;
#107995=AXIS2_PLACEMENT_3D ( 'NONE', #105114, #113659, #15435 ) ;
#108045=DIRECTION ( 'NONE',  ( 0.000000000000000000, 1.846105847067148761E-16, 1.000000000000000000 ) ) ;
#108077=ORIENTED_EDGE ( 'NONE', *, *, #43595, .T. ) ;
#108094=DIRECTION ( 'NONE',  ( -1.000000000000000000, -0.000000000000000000, -0.000000000000000000 ) ) ;
#108100=VECTOR ( 'NONE', #65026, 1000.000000000000000 ) ;
#108134=CARTESIAN_POINT ( 'NONE',  ( 184.7083333333333144, -4.445597072760115509, -7.700000000000001954 ) ) ;
#108172=DIRECTION ( 'NONE',  ( 0.000000000000000000, -1.846105847067148515E-16, -1.000000000000000000 ) ) ;
#108173=CARTESIAN_POINT ( 'NONE',  ( 186.8593750003414016, 0.000000000000000000, 7.564683531250000925 ) ) ;
#108175=CARTESIAN_POINT ( 'NONE',  ( 104.0348890100390946, 8.147879001971702451, 3.062904332527759621 ) ) ;
#108257=CARTESIAN_POINT ( 'NONE',  ( 112.3243458019354648, 8.328603270140316539, -2.530626142253337374 ) ) ;
#108267=ADVANCED_FACE ( 'NONE', ( #74170 ), #12647, .T. ) ;
#108296=AXIS2_PLACEMENT_3D ( 'NONE', #10644, #90516, #80718 ) ;
#108357=EDGE_CURVE ( 'NONE', #115280, #60931, #31926, .T. ) ;
#108380=CARTESIAN_POINT ( 'NONE',  ( 185.3593750003413732, 0.000000000000000000, 7.564683531250000925 ) ) ;
#108408=DIRECTION ( 'NONE',  ( 0.000000000000000000, 0.000000000000000000, -1.000000000000000000 ) ) ;
#108489=CARTESIAN_POINT ( 'NONE',  ( 186.0052083336747444, -6.551208109652278289, 3.782341765624995134 ) ) ;
#108536=ORIENTED_EDGE ( 'NONE', *, *, #116320, .T. ) ;
#108546=CARTESIAN_POINT ( 'NONE',  ( 108.6775537376563534, 5.892458298213239409, 4.956757361901918735 ) ) ;
#108583=CARTESIAN_POINT ( 'NONE',  ( 185.9843750003414016, -8.734944146203032389, -1.604583208406768146E-15 ) ) ;
#108665=PLANE ( 'NONE',  #115559 ) ;
#108684=CARTESIAN_POINT ( 'NONE',  ( 184.5312500006828031, 9.429780353434619030E-16, -7.700000000000000178 ) ) ;
#108692=VECTOR ( 'NONE', #77379, 1000.000000000000000 ) ;
#108813=CARTESIAN_POINT ( 'NONE',  ( 186.0312500006828031, 9.429780353434619030E-16, -7.700000000000000178 ) ) ;
#108815=CARTESIAN_POINT ( 'NONE',  ( 103.0003941427382301, 8.699773481286413812, 0.3429536323214144589 ) ) ;
#109010=CARTESIAN_POINT ( 'NONE',  ( 184.7760416670080588, 6.551208109652274736, 3.782341765625001351 ) ) ;
#109027=CARTESIAN_POINT ( 'NONE',  ( 179.5000000000000000, 1.375000000000000222, 6.000000000000000000 ) ) ;
#109029=CIRCLE ( 'NONE', #52606, 8.699999999999999289 ) ;
#109031=CARTESIAN_POINT ( 'NONE',  ( 184.5000000000000000, 0.000000000000000000, 7.700000000000000178 ) ) ;
#109041=VERTEX_POINT ( 'NONE', #61949 ) ;
#109141=ADVANCED_FACE ( 'NONE', ( #92687 ), #93977, .T. ) ;
#109212=CARTESIAN_POINT ( 'NONE',  ( 186.9010416670080303, -4.367472073101519747, 7.564683531249999149 ) ) ;
#109361=SHAPE_REPRESENTATION_RELATIONSHIP ( 'NONE' , 'NONE' ,  #5058, #78940 ) ;
#109391=FACE_OUTER_BOUND ( 'NONE', #60958, .T. ) ;
#109437=DIRECTION ( 'NONE',  ( -1.000000000000000000, -0.000000000000000000, -0.000000000000000000 ) ) ;
#109474=LINE ( 'NONE', #78083, #6995 ) ;
#109540=EDGE_LOOP ( 'NONE', ( #71463, #58683, #19118, #46349 ) ) ;
#109586=ORIENTED_EDGE ( 'NONE', *, *, #42622, .F. ) ;
#109625=VERTEX_POINT ( 'NONE', #55193 ) ;
#109628=CARTESIAN_POINT ( 'NONE',  ( 183.7812500006828031, 0.000000000000000000, 7.700000000000000178 ) ) ;
#109681=CARTESIAN_POINT ( 'NONE',  ( 186.2343750003414016, 8.734944146203032389, 5.348610694689227483E-16 ) ) ;
#109682=DIRECTION ( 'NONE',  ( -1.000000000000000000, 0.000000000000000000, 0.000000000000000000 ) ) ;
#109727=CYLINDRICAL_SURFACE ( 'NONE', #39681, 7.700000000000000178 ) ;
#109880=CARTESIAN_POINT ( 'NONE',  ( 185.8177083336747444, 4.367472073101515306, 7.564683531250000925 ) ) ;
#109973=CYLINDRICAL_SURFACE ( 'NONE', #11448, 7.700000000000000178 ) ;
#109999=DIRECTION ( 'NONE',  ( 0.000000000000000000, -1.000000000000000000, -0.000000000000000000 ) ) ;
#110046=CARTESIAN_POINT ( 'NONE',  ( 186.4583333333333428, 4.445597072760147483, 7.699999999999948663 ) ) ;
#110091=ORIENTED_EDGE ( 'NONE', *, *, #101185, .T. ) ;
#110227=CARTESIAN_POINT ( 'NONE',  ( 187.2135416670080588, 4.367472073101518859, -7.564683531249999149 ) ) ;
#110244=ORIENTED_EDGE ( 'NONE', *, *, #23025, .F. ) ;
#110288=AXIS2_PLACEMENT_3D ( 'NONE', #16128, #126100, #73776 ) ;
#110318=EDGE_CURVE ( 'NONE', #97447, #31133, #100740, .T. ) ;
#110319=CARTESIAN_POINT ( 'NONE',  ( 184.2760416670080588, 6.551208109652274736, 3.782341765625001351 ) ) ;
#110333=AXIS2_PLACEMENT_3D ( 'NONE', #23575, #19210, #98414 ) ;
#110374=AXIS2_PLACEMENT_3D ( 'NONE', #32868, #72770, #3379 ) ;
#110378=VERTEX_POINT ( 'NONE', #9799 ) ;
#110448=VECTOR ( 'NONE', #85694, 1000.000000000000000 ) ;
#110456=CARTESIAN_POINT ( 'NONE',  ( 129.5000000000000000, 0.000000000000000000, 7.700000000000000178 ) ) ;
#110515=CARTESIAN_POINT ( 'NONE',  ( 187.3593750003414016, 0.000000000000000000, 7.564683531250000925 ) ) ;
#110591=PLANE ( 'NONE',  #85845 ) ;
#110633=LINE ( 'NONE', #40638, #97746 ) ;
#110641=CARTESIAN_POINT ( 'NONE',  ( 103.6920052614127030, 7.269452028459965298, 2.543125990730006336 ) ) ;
#110705=CARTESIAN_POINT ( 'NONE',  ( 184.0000000000000000, 0.000000000000000000, 7.700000000000000178 ) ) ;
#110717=EDGE_CURVE ( 'NONE', #43268, #2171, #66622, .T. ) ;
#110751=CARTESIAN_POINT ( 'NONE',  ( 185.9010416670080303, -4.367472073101520635, 7.564683531249999149 ) ) ;
#110841=CARTESIAN_POINT ( 'NONE',  ( 127.5000000000000000, -1.500000000000000000, -2.598076211353316900 ) ) ;
#110846=ORIENTED_EDGE ( 'NONE', *, *, #39742, .F. ) ;
#110854=CARTESIAN_POINT ( 'NONE',  ( 187.0468750003414300, -8.734944146203032389, -1.604583208406768146E-15 ) ) ;
#111056=VERTEX_POINT ( 'NONE', #46677 ) ;
#111137=CARTESIAN_POINT ( 'NONE',  ( 184.9010416670080588, -4.367472073101519747, 7.564683531249999149 ) ) ;
#111158=DIRECTION ( 'NONE',  ( 0.000000000000000000, 0.000000000000000000, -1.000000000000000000 ) ) ;
#111172=VERTEX_POINT ( 'NONE', #97063 ) ;
#111208=CARTESIAN_POINT ( 'NONE',  ( 129.5000000000000000, -1.375000000000000000, 7.634788798650553154 ) ) ;
#111305=AXIS2_PLACEMENT_3D ( 'NONE', #57295, #8177, #38305 ) ;
#111321=VECTOR ( 'NONE', #83147, 1000.000000000000000 ) ;
#111386=CARTESIAN_POINT ( 'NONE',  ( 184.7343750003414016, 8.734944146203032389, 5.348610694689227483E-16 ) ) ;
#111508=CARTESIAN_POINT ( 'NONE',  ( 186.9218750003414016, 0.000000000000000000, 7.564683531250000925 ) ) ;
#111532=ORIENTED_EDGE ( 'NONE', *, *, #39747, .T. ) ;
#111619=EDGE_CURVE ( 'NONE', #74365, #7606, #66151, .T. ) ;
#111764=CARTESIAN_POINT ( 'NONE',  ( 186.8229166673494319, -4.445597072760122614, 7.699999999999998401 ) ) ;
#111802=CYLINDRICAL_SURFACE ( 'NONE', #53268, 7.700000000000000178 ) ;
#111817=CARTESIAN_POINT ( 'NONE',  ( 186.2552083336747444, 6.551208109652275624, -3.782341765624998686 ) ) ;
#111904=CARTESIAN_POINT ( 'NONE',  ( 186.6562500006828031, 8.891194145520236347, 5.444286225454521982E-16 ) ) ;
#111936=ORIENTED_EDGE ( 'NONE', *, *, #97903, .F. ) ;
#112058=CARTESIAN_POINT ( 'NONE',  ( 184.9843750003414016, -8.734944146203032389, -1.604583208406767949E-15 ) ) ;
#112135=VECTOR ( 'NONE', #68184, 1000.000000000000000 ) ;
#112160=ORIENTED_EDGE ( 'NONE', *, *, #10204, .T. ) ;
#112208=CARTESIAN_POINT ( 'NONE',  ( 129.5000000000000000, -0.6250000000000000000, 7.634788798650553154 ) ) ;
#112266=EDGE_CURVE ( 'NONE', #48297, #41599, #39431, .T. ) ;
#112311=LINE ( 'NONE', #63852, #32262 ) ;
#112317=ORIENTED_EDGE ( 'NONE', *, *, #125392, .T. ) ;
#112330=ORIENTED_EDGE ( 'NONE', *, *, #20926, .T. ) ;
#112347=CARTESIAN_POINT ( 'NONE',  ( 127.5000000000000000, 0.000000000000000000, 0.000000000000000000 ) ) ;
#112354=ORIENTED_EDGE ( 'NONE', *, *, #11245, .F. ) ;
#112399=CIRCLE ( 'NONE', #55951, 8.199999999999999289 ) ;
#112464=CARTESIAN_POINT ( 'NONE',  ( 186.2135416670080872, 4.367472073101518859, -7.564683531249999149 ) ) ;
#112483=PLANE ( 'NONE',  #79990 ) ;
#112539=EDGE_CURVE ( 'NONE', #8359, #16632, #91406, .T. ) ;
#112565=CARTESIAN_POINT ( 'NONE',  ( 186.9895833340161744, -4.445597072760123503, -7.699999999999989519 ) ) ;
#112599=CARTESIAN_POINT ( 'NONE',  ( 184.8645833340161175, -6.668395609140180369, 3.849999999999994760 ) ) ;
#112617=AXIS2_PLACEMENT_3D ( 'NONE', #112347, #122809, #63886 ) ;
#112703=CARTESIAN_POINT ( 'NONE',  ( 183.8593750003413732, 0.000000000000000000, 7.564683531250000925 ) ) ;
#112811=CARTESIAN_POINT ( 'NONE',  ( 184.6302083336747444, -4.367472073101514418, -7.564683531250002702 ) ) ;
#112872=DIRECTION ( 'NONE',  ( 0.000000000000000000, 0.000000000000000000, -1.000000000000000000 ) ) ;
#112951=DIRECTION ( 'NONE',  ( 1.000000000000000000, 0.000000000000000000, 0.000000000000000000 ) ) ;
#112987=CARTESIAN_POINT ( 'NONE',  ( 186.4479166673494603, -6.668395609140176816, -3.850000000000003642 ) ) ;
#113042=CARTESIAN_POINT ( 'NONE',  ( 186.9895833340161460, -4.445597072760115509, -7.700000000000001954 ) ) ;
#113077=DIRECTION ( 'NONE',  ( -1.000000000000000000, -0.000000000000000000, -0.000000000000000000 ) ) ;
#113087=CARTESIAN_POINT ( 'NONE',  ( 186.9635416670080303, -4.367472073101519747, 7.564683531249999149 ) ) ;
#113208=CARTESIAN_POINT ( 'NONE',  ( 103.2667551388651930, 7.528838585660450278, -1.644710558206996964 ) ) ;
#113247=CARTESIAN_POINT ( 'NONE',  ( 112.3254613740535177, 8.329167917205943183, 2.528930095568325598 ) ) ;
#113331=CARTESIAN_POINT ( 'NONE',  ( 185.3593750003413732, 0.000000000000000000, 7.564683531250000925 ) ) ;
#113403=CARTESIAN_POINT ( 'NONE',  ( 183.8906250003414016, 0.000000000000000000, 7.700000000000000178 ) ) ;
#113446=CARTESIAN_POINT ( 'NONE',  ( 185.4635416670080872, -4.367472073101519747, 7.564683531249999149 ) ) ;
#113538=DIRECTION ( 'NONE',  ( 0.000000000000000000, 0.000000000000000000, -1.000000000000000000 ) ) ;
#113552=ORIENTED_EDGE ( 'NONE', *, *, #35659, .T. ) ;
#113580=VERTEX_POINT ( 'NONE', #3991 ) ;
#113603=CARTESIAN_POINT ( 'NONE',  ( 187.5000000000000000, 9.429780353434619030E-16, -7.700000000000000178 ) ) ;
#113659=DIRECTION ( 'NONE',  ( 1.000000000000000000, 0.000000000000000000, 0.000000000000000000 ) ) ;
#113699=CARTESIAN_POINT ( 'NONE',  ( 185.4895833340161175, -4.445597072760115509, -7.700000000000001954 ) ) ;
#113742=ORIENTED_EDGE ( 'NONE', *, *, #50030, .T. ) ;
#113750=CARTESIAN_POINT ( 'NONE',  ( 184.6510416670080588, 4.367472073101518859, -7.564683531249999149 ) ) ;
#113872=CARTESIAN_POINT ( 'NONE',  ( 104.0411730856320389, 7.066873072444588288, -3.070937804656772130 ) ) ;
#113920=ADVANCED_FACE ( 'NONE', ( #35262 ), #22870, .F. ) ;
#113968=CARTESIAN_POINT ( 'NONE',  ( 179.5000000000000000, 1.375000000000000000, 7.634788798650556707 ) ) ;
#113984=EDGE_CURVE ( 'NONE', #102067, #14892, #871, .T. ) ;
#114057=DIRECTION ( 'NONE',  ( 1.000000000000000000, -0.000000000000000000, -0.000000000000000000 ) ) ;
#114094=CARTESIAN_POINT ( 'NONE',  ( 185.8802083336747444, 4.367472073101515306, 7.564683531250000925 ) ) ;
#114108=ORIENTED_EDGE ( 'NONE', *, *, #96435, .F. ) ;
#114147=ADVANCED_FACE ( 'NONE', ( #82268 ), #73081, .F. ) ;
#114186=AXIS2_PLACEMENT_3D ( 'NONE', #12640, #124552, #42791 ) ;
#114215=LINE ( 'NONE', #76231, #69991 ) ;
#114300=VERTEX_POINT ( 'NONE', #56638 ) ;
#114371=CARTESIAN_POINT ( 'NONE',  ( 184.1302083336747160, -4.367472073101514418, -7.564683531250002702 ) ) ;
#114388=ORIENTED_EDGE ( 'NONE', *, *, #10553, .T. ) ;
#114411=DIRECTION ( 'NONE',  ( -1.000000000000000000, -0.000000000000000000, -0.000000000000000000 ) ) ;
#114441=CARTESIAN_POINT ( 'NONE',  ( 186.8802083336747444, 4.367472073101515306, 7.564683531250000925 ) ) ;
#114480=CARTESIAN_POINT ( 'NONE',  ( 186.7812500006828031, 0.000000000000000000, 7.700000000000000178 ) ) ;
#114625=VERTEX_POINT ( 'NONE', #62482 ) ;
#114709=ADVANCED_FACE ( 'NONE', ( #84677 ), #108665, .F. ) ;
#114730=CARTESIAN_POINT ( 'NONE',  ( 184.7552083336747444, 6.551208109652275624, -3.782341765624998686 ) ) ;
#114754=CARTESIAN_POINT ( 'NONE',  ( 186.5416666666666572, -4.445597072760092416, 7.700000000000049916 ) ) ;
#114828=VERTEX_POINT ( 'NONE', #22884 ) ;
#114932=EDGE_LOOP ( 'NONE', ( #85544, #119324, #3422, #91862 ) ) ;
#114937=DIRECTION ( 'NONE',  ( 0.000000000000000000, -1.846105847067148022E-16, 1.000000000000000000 ) ) ;
#114963=CARTESIAN_POINT ( 'NONE',  ( 184.7812500006828031, 0.000000000000000000, 7.700000000000000178 ) ) ;
#115072=CYLINDRICAL_SURFACE ( 'NONE', #21729, 7.700000000000000178 ) ;
#115199=EDGE_CURVE ( 'NONE', #92765, #44902, #49617, .T. ) ;
#115265=CARTESIAN_POINT ( 'NONE',  ( 185.7500000000000000, 9.429780353434619030E-16, -7.700000000000000178 ) ) ;
#115280=VERTEX_POINT ( 'NONE', #29111 ) ;
#115290=CARTESIAN_POINT ( 'NONE',  ( 179.5000000000000000, 0.6250000000000028866, -7.634788798650556707 ) ) ;
#115302=CARTESIAN_POINT ( 'NONE',  ( 185.0000000000000000, 0.000000000000000000, 7.700000000000000178 ) ) ;
#115331=AXIS2_PLACEMENT_3D ( 'NONE', #51882, #91797, #42058 ) ;
#115339=EDGE_CURVE ( 'NONE', #66080, #97447, #76901, .T. ) ;
#115351=CARTESIAN_POINT ( 'NONE',  ( 185.0052083336747444, -6.551208109652278289, 3.782341765624995134 ) ) ;
#115420=EDGE_CURVE ( 'NONE', #122603, #114300, #87346, .T. ) ;
#115448=DIRECTION ( 'NONE',  ( 1.000000000000000000, 0.000000000000000000, 0.000000000000000000 ) ) ;
#115559=AXIS2_PLACEMENT_3D ( 'NONE', #58297, #18986, #98200 ) ;
#115610=CARTESIAN_POINT ( 'NONE',  ( 186.5260416670080588, -6.551208109652273848, -3.782341765625003571 ) ) ;
#115656=CARTESIAN_POINT ( 'NONE',  ( 184.9635416670080872, -4.367472073101519747, 7.564683531249999149 ) ) ;
#115661=EDGE_CURVE ( 'NONE', #129597, #109041, #4120, .T. ) ;
#115730=CARTESIAN_POINT ( 'NONE',  ( 186.3802083336747444, 4.367472073101515306, 7.564683531250000925 ) ) ;
#115849=CARTESIAN_POINT ( 'NONE',  ( 187.0729166673494603, 4.445597072760113733, -7.700000000000009948 ) ) ;
#115947=DIRECTION ( 'NONE',  ( 0.000000000000000000, -1.000000000000000000, 0.000000000000000000 ) ) ;
#116007=EDGE_CURVE ( 'NONE', #55407, #19872, #114215, .T. ) ;
#116019=CARTESIAN_POINT ( 'NONE',  ( 185.7500000000000000, 9.429780353434619030E-16, -7.700000000000000178 ) ) ;
#116057=DIRECTION ( 'NONE',  ( -1.000000000000000000, -0.000000000000000000, -0.000000000000000000 ) ) ;
#116111=PRODUCT_DEFINITION_CONTEXT ( 'detailed design', #125709, 'design' ) ;
#116140=CARTESIAN_POINT ( 'NONE',  ( 108.6700850095774626, 7.143942430811406119, -4.965926407314869451 ) ) ;
#116188=VERTEX_POINT ( 'NONE', #121301 ) ;
#116259=CARTESIAN_POINT ( 'NONE',  ( 183.9479166673494603, -6.668395609140176816, -3.850000000000003642 ) ) ;
#116267=AXIS2_PLACEMENT_3D ( 'NONE', #98869, #68116, #108045 ) ;
#116297=CARTESIAN_POINT ( 'NONE',  ( 185.0468750003414016, -8.734944146203032389, -1.604583208406768146E-15 ) ) ;
#116316=ORIENTED_EDGE ( 'NONE', *, *, #43250, .T. ) ;
#116319=LINE ( 'NONE', #16813, #73090 ) ;
#116320=EDGE_CURVE ( 'NONE', #15804, #97447, #101013, .T. ) ;
#116371=CARTESIAN_POINT ( 'NONE',  ( 184.5468750003414300, -8.734944146203032389, -1.604583208406767949E-15 ) ) ;
#116510=EDGE_CURVE ( 'NONE', #119603, #4736, #90877, .T. ) ;
#116663=CARTESIAN_POINT ( 'NONE',  ( 184.5833333333333144, -6.668395609140180369, 3.849999999999994760 ) ) ;
#116695=COLOUR_RGB ( '', 0.40784314, 0.44705882, 0.49803922) ;
#116857=CARTESIAN_POINT ( 'NONE',  ( 184.7500000000000000, 9.429780353434619030E-16, -7.700000000000000178 ) ) ;
#116895=CARTESIAN_POINT ( 'NONE',  ( 184.1979166673494603, 6.668395609140176816, 3.850000000000000977 ) ) ;
#116911=CARTESIAN_POINT ( 'NONE',  ( 179.5000000000000000, 0.6250000000000000000, 7.634788798650556707 ) ) ;
#116939=CARTESIAN_POINT ( 'NONE',  ( 184.6302083336747444, -4.367472073101514418, -7.564683531250002702 ) ) ;
#117004=CARTESIAN_POINT ( 'NONE',  ( 186.2552083336747444, 6.551208109652275624, -3.782341765624998686 ) ) ;
#117106=VERTEX_POINT ( 'NONE', #63850 ) ;
#117119=ORIENTED_EDGE ( 'NONE', *, *, #25318, .F. ) ;
#117177=AXIS2_PLACEMENT_3D ( 'NONE', #71390, #41960, #72071 ) ;
#117278=CARTESIAN_POINT ( 'NONE',  ( 186.7916666666666572, 4.445597072760120838, -7.699999999999998401 ) ) ;
#117285=DIRECTION ( 'NONE',  ( 0.000000000000000000, 0.000000000000000000, 1.000000000000000000 ) ) ;
#117323=DIRECTION ( 'NONE',  ( 0.000000000000000000, 0.000000000000000000, -1.000000000000000000 ) ) ;
#117324=AXIS2_PLACEMENT_3D ( 'NONE', #57062, #70760, #4404 ) ;
#117359=ORIENTED_EDGE ( 'NONE', *, *, #14550, .F. ) ;
#117402=CARTESIAN_POINT ( 'NONE',  ( 186.1250000000000000, -8.891194145520236347, -1.633285867636356299E-15 ) ) ;
#117404=CARTESIAN_POINT ( 'NONE',  ( 108.3389004593042415, 7.119691004531022216, -5.000000000000006217 ) ) ;
#117429=ORIENTED_EDGE ( 'NONE', *, *, #43347, .F. ) ;
#117435=CARTESIAN_POINT ( 'NONE',  ( 179.5000000000000000, 0.6250000000000028866, -7.634788798650556707 ) ) ;
#117465=ORIENTED_EDGE ( 'NONE', *, *, #110717, .F. ) ;
#117479=CARTESIAN_POINT ( 'NONE',  ( 184.8333333333333144, 6.668395609140177704, -3.849999999999998312 ) ) ;
#117517=CARTESIAN_POINT ( 'NONE',  ( 129.5000000000000000, -0.6250000000000000000, 7.634788798650553154 ) ) ;
#117528=CARTESIAN_POINT ( 'NONE',  ( 184.0729166673494603, 4.445597072760120838, -7.699999999999998401 ) ) ;
#117642=CARTESIAN_POINT ( 'NONE',  ( 184.3385416670080872, 6.551208109652274736, 3.782341765625001351 ) ) ;
#117734=CARTESIAN_POINT ( 'NONE',  ( 186.9427083336747160, -6.551208109652278289, 3.782341765624995134 ) ) ;
#117750=ORIENTED_EDGE ( 'NONE', *, *, #86612, .F. ) ;
#117773=CARTESIAN_POINT ( 'NONE',  ( 179.5000000000000000, 0.000000000000000000, 6.000000000000000000 ) ) ;
#117790=VECTOR ( 'NONE', #98102, 1000.000000000000000 ) ;
#117865=LINE ( 'NONE', #97591, #94610 ) ;
#117867=DIRECTION ( 'NONE',  ( -1.000000000000000000, -0.000000000000000000, -0.000000000000000000 ) ) ;
#117932=CARTESIAN_POINT ( 'NONE',  ( 179.5000000000000000, -0.6250000000000028866, -7.634788798650553154 ) ) ;
#117946=CARTESIAN_POINT ( 'NONE',  ( 186.7500000000000000, 9.429780353434619030E-16, -7.700000000000000178 ) ) ;
#117968=ORIENTED_EDGE ( 'NONE', *, *, #104968, .F. ) ;
#117995=CARTESIAN_POINT ( 'NONE',  ( 187.1927083336747160, 6.551208109652275624, -3.782341765624998686 ) ) ;
#118008=ORIENTED_EDGE ( 'NONE', *, *, #126703, .F. ) ;
#118032=ORIENTED_EDGE ( 'NONE', *, *, #42804, .F. ) ;
#118154=EDGE_LOOP ( 'NONE', ( #85585, #46253, #105626, #30020, #11380, #21460, #53421, #90818 ) ) ;
#118182=CARTESIAN_POINT ( 'NONE',  ( 186.2500000000000000, 9.429780353434619030E-16, -7.700000000000000178 ) ) ;
#118204=CARTESIAN_POINT ( 'NONE',  ( 185.8593750003413732, 0.000000000000000000, 7.564683531250000925 ) ) ;
#118313=CARTESIAN_POINT ( 'NONE',  ( 185.8802083336747444, 4.367472073101515306, 7.564683531250000925 ) ) ;
#118320=VECTOR ( 'NONE', #96248, 1000.000000000000000 ) ;
#118358=CARTESIAN_POINT ( 'NONE',  ( 112.9991567705375388, 7.699452449333159976, -0.3520876866445218356 ) ) ;
#118393=CARTESIAN_POINT ( 'NONE',  ( 129.5000000000000000, 0.000000000000000000, 6.000000000000000000 ) ) ;
#118397=CARTESIAN_POINT ( 'NONE',  ( 186.5260416670080588, -6.551208109652273848, -3.782341765625003571 ) ) ;
#118494=VECTOR ( 'NONE', #119245, 1000.000000000000000 ) ;
#118515=DIRECTION ( 'NONE',  ( 0.000000000000000000, 1.000000000000000000, 0.000000000000000000 ) ) ;
#118533=CARTESIAN_POINT ( 'NONE',  ( 185.9166666666666856, 6.668395609140176816, 3.850000000000000977 ) ) ;
#118596=CARTESIAN_POINT ( 'NONE',  ( 184.3333333333333144, 6.668395609140177704, -3.849999999999998312 ) ) ;
#118610=( BOUNDED_CURVE ( )  B_SPLINE_CURVE ( 2, ( #126810, #48244, #107151, #88139, #128098, #17475, #38446 ),
 .UNSPECIFIED., .F., .F. ) 
 B_SPLINE_CURVE_WITH_KNOTS ( ( 3, 2, 2, 3 ),
 ( 0.5714285714285719520, 0.5952380952380957879, 0.6190476190476195129, 0.6428571428571433488 ),
 .UNSPECIFIED. ) 
 CURVE ( )  GEOMETRIC_REPRESENTATION_ITEM ( )  RATIONAL_B_SPLINE_CURVE ( ( 0.9999999999999968914, 0.8660254037844418162, 1.000000000000000000, 0.8660254037844387076, 1.000000000000000000, 0.8660254037844361541, 1.000000000000002442 ) ) 
 REPRESENTATION_ITEM ( '' )  );
#118624=CARTESIAN_POINT ( 'NONE',  ( 185.4479166673494603, -6.668395609140176816, -3.850000000000003642 ) ) ;
#118639=CIRCLE ( 'NONE', #99782, 8.199999999999999289 ) ;
#118665=CARTESIAN_POINT ( 'NONE',  ( 129.5000000000000000, 1.500000000000000000, 2.598076211353316900 ) ) ;
#118671=CIRCLE ( 'NONE', #89344, 7.700000000000000178 ) ;
#118675=CIRCLE ( 'NONE', #70655, 8.699999999999999289 ) ;
#118755=EDGE_CURVE ( 'NONE', #114828, #114625, #97624, .T. ) ;
#118845=CARTESIAN_POINT ( 'NONE',  ( 184.4427083336747160, -6.551208109652278289, 3.782341765624995134 ) ) ;
#118850=VERTEX_POINT ( 'NONE', #38278 ) ;
#119020=ADVANCED_FACE ( 'NONE', ( #15226 ), #7348, .F. ) ;
#119054=CARTESIAN_POINT ( 'NONE',  ( 185.9427083336747160, -6.551208109652278289, 3.782341765624995134 ) ) ;
#119086=EDGE_LOOP ( 'NONE', ( #87695, #29424 ) ) ;
#119175=CARTESIAN_POINT ( 'NONE',  ( 106.6738984060675079, 6.002110804423450574, 4.823747364179781449 ) ) ;
#119245=DIRECTION ( 'NONE',  ( 0.000000000000000000, -1.000000000000000000, 0.000000000000000000 ) ) ;
#119265=CARTESIAN_POINT ( 'NONE',  ( 185.4895833340161175, -4.445597072760163471, -7.699999999999919353 ) ) ;
#119285=CARTESIAN_POINT ( 'NONE',  ( 186.4010416670080588, -4.367472073101520635, 7.564683531249999149 ) ) ;
#119288=CARTESIAN_POINT ( 'NONE',  ( 105.7595978339907390, 7.458259062902370395, 4.481802286990411055 ) ) ;
#119289=DIRECTION ( 'NONE',  ( 0.000000000000000000, -1.000000000000000000, 0.000000000000000000 ) ) ;
#119324=ORIENTED_EDGE ( 'NONE', *, *, #43595, .F. ) ;
#119381=CARTESIAN_POINT ( 'NONE',  ( 184.1979166673494603, 6.668395609140176816, 3.850000000000000977 ) ) ;
#119391=DIRECTION ( 'NONE',  ( -1.000000000000000000, 0.000000000000000000, 0.000000000000000000 ) ) ;
#119465=ORIENTED_EDGE ( 'NONE', *, *, #912, .F. ) ;
#119482=CARTESIAN_POINT ( 'NONE',  ( 185.9843750003414016, -8.734944146203032389, -1.604583208406768146E-15 ) ) ;
#119553=ORIENTED_EDGE ( 'NONE', *, *, #36681, .F. ) ;
#119555=ORIENTED_EDGE ( 'NONE', *, *, #90954, .T. ) ;
#119603=VERTEX_POINT ( 'NONE', #14214 ) ;
#119680=CARTESIAN_POINT ( 'NONE',  ( 185.5677083336747160, -4.367472073101514418, -7.564683531250002702 ) ) ;
#119781=DIRECTION ( 'NONE',  ( 0.000000000000000000, 1.000000000000000000, 0.000000000000000000 ) ) ;
#119786=CARTESIAN_POINT ( 'NONE',  ( 185.6979166673494603, 6.668395609140176816, 3.850000000000000977 ) ) ;
#119895=CARTESIAN_POINT ( 'NONE',  ( 184.2083333333333144, -4.445597072760115509, -7.700000000000001954 ) ) ;
#119942=CARTESIAN_POINT ( 'NONE',  ( 187.1510416670080588, 4.367472073101518859, -7.564683531249999149 ) ) ;
#119946=CARTESIAN_POINT ( 'NONE',  ( 103.0665022457567943, 8.661908772191825534, -0.8295545705914831869 ) ) ;
#120022=CARTESIAN_POINT ( 'NONE',  ( 110.2387336715401318, 7.457814704407476292, 4.482516261046311179 ) ) ;
#120051=CARTESIAN_POINT ( 'NONE',  ( 186.7968750003414300, 8.734944146203032389, 5.348610694689227483E-16 ) ) ;
#120143=CARTESIAN_POINT ( 'NONE',  ( 184.5260416670080588, -6.551208109652273848, -3.782341765625003571 ) ) ;
#120293=VECTOR ( 'NONE', #73085, 1000.000000000000000 ) ;
#120331=CARTESIAN_POINT ( 'NONE',  ( 185.5833333333333144, -6.668395609140180369, 3.849999999999994760 ) ) ;
#120347=CARTESIAN_POINT ( 'NONE',  ( 187.1093750003414016, 9.264065473108010111E-16, -7.564683531250000925 ) ) ;
#120379=EDGE_LOOP ( 'NONE', ( #65341, #95235, #117968, #107978 ) ) ;
#120433=CARTESIAN_POINT ( 'NONE',  ( 186.6979166673494603, 6.668395609140176816, 3.850000000000000977 ) ) ;
#120458=DIRECTION ( 'NONE',  ( -1.000000000000000000, 0.000000000000000000, 0.000000000000000000 ) ) ;
#120465=CARTESIAN_POINT ( 'NONE',  ( 104.2474658290071687, 6.952256801654628227, 3.319715706849921677 ) ) ;
#120586=CARTESIAN_POINT ( 'NONE',  ( 103.2667367461191077, 8.548823231429411251, 1.644105246313542157 ) ) ;
#120605=CARTESIAN_POINT ( 'NONE',  ( 186.5000000000000000, 0.000000000000000000, 7.700000000000000178 ) ) ;
#120666=CARTESIAN_POINT ( 'NONE',  ( 109.1593346011806887, 7.211655450534177447, 4.866583586154797025 ) ) ;
#120691=CARTESIAN_POINT ( 'NONE',  ( 186.8385416670080872, 6.551208109652274736, 3.782341765625001351 ) ) ;
#120759=CYLINDRICAL_SURFACE ( 'NONE', #61688, 7.700000000000000178 ) ;
#120928=DIRECTION ( 'NONE',  ( 1.000000000000000000, 0.000000000000000000, 0.000000000000000000 ) ) ;
#120982=CARTESIAN_POINT ( 'NONE',  ( 187.2135416670080588, 4.367472073101518859, -7.564683531249999149 ) ) ;
#121004=FACE_OUTER_BOUND ( 'NONE', #119086, .T. ) ;
#121020=AXIS2_PLACEMENT_3D ( 'NONE', #73604, #115448, #113538 ) ;
#121046=CARTESIAN_POINT ( 'NONE',  ( 184.0416666666666572, -4.445597072760122614, 7.699999999999997513 ) ) ;
#121048=ORIENTED_EDGE ( 'NONE', *, *, #71695, .F. ) ;
#121068=VERTEX_POINT ( 'NONE', #109031 ) ;
#121224=CARTESIAN_POINT ( 'NONE',  ( 184.4010416670081156, -4.367472073101520635, 7.564683531249999149 ) ) ;
#121272=DIRECTION ( 'NONE',  ( 0.000000000000000000, 1.846105847067148022E-16, -1.000000000000000000 ) ) ;
#121289=( BOUNDED_CURVE ( )  B_SPLINE_CURVE ( 2, ( #17032, #39950, #119786, #106732, #7236, #47191, #123018 ),
 .UNSPECIFIED., .F., .F. ) 
 B_SPLINE_CURVE_WITH_KNOTS ( ( 3, 2, 2, 3 ),
 ( 0.4285714285714289362, 0.4523809523809527722, 0.4761904761904766081, 0.5000000000000004441 ),
 .UNSPECIFIED. ) 
 CURVE ( )  GEOMETRIC_REPRESENTATION_ITEM ( )  RATIONAL_B_SPLINE_CURVE ( ( 0.9999999999999977796, 0.8660254037844409281, 1.000000000000000000, 0.8660254037844387076, 1.000000000000000000, 0.8660254037844361541, 1.000000000000002442 ) ) 
 REPRESENTATION_ITEM ( '' )  );
#121301=CARTESIAN_POINT ( 'NONE',  ( 187.0312500006828031, 9.429780353434619030E-16, -7.700000000000000178 ) ) ;
#121413=EDGE_LOOP ( 'NONE', ( #34793, #69212, #76669, #27593, #47937, #100075, #109586, #73548, #49194, #75825, #106386, #22270, #29491, #10414, #119553, #33284, #11594 ) ) ;
#121464=CARTESIAN_POINT ( 'NONE',  ( 187.5000000000000000, 0.000000000000000000, 0.000000000000000000 ) ) ;
#121565=CARTESIAN_POINT ( 'NONE',  ( 186.4479166673494603, -6.668395609140176816, -3.850000000000003642 ) ) ;
#121612=CARTESIAN_POINT ( 'NONE',  ( 183.8593750003413732, 0.000000000000000000, 7.564683531250000925 ) ) ;
#121784=CYLINDRICAL_SURFACE ( 'NONE', #117177, 7.700000000000000178 ) ;
#121868=CARTESIAN_POINT ( 'NONE',  ( 185.6510416670080303, 4.367472073101518859, -7.564683531249999149 ) ) ;
#121906=ADVANCED_FACE ( 'NONE', ( #68656 ), #84584, .F. ) ;
#122064=( BOUNDED_CURVE ( )  B_SPLINE_CURVE ( 2, ( #61824, #11412, #22548, #40238, #29769, #72288, #109628 ),
 .UNSPECIFIED., .F., .T. ) 
 B_SPLINE_CURVE_WITH_KNOTS ( ( 3, 2, 2, 3 ),
 ( 0.9285714285714292693, 0.9523809523809527722, 0.9761904761904763861, 1.000000000000000000 ),
 .UNSPECIFIED. ) 
 CURVE ( )  GEOMETRIC_REPRESENTATION_ITEM ( )  RATIONAL_B_SPLINE_CURVE ( ( 0.9999999999999962252, 0.8660254037844424824, 1.000000000000000000, 0.8660254037844387076, 1.000000000000000000, 0.8660254037844387076, 1.000000000000000000 ) ) 
 REPRESENTATION_ITEM ( '' )  );
#122238=CARTESIAN_POINT ( 'NONE',  ( 186.6562500006828316, 8.891194145520236347, 5.444286225454521982E-16 ) ) ;
#122277=ADVANCED_FACE ( 'NONE', ( #55317 ), #34406, .F. ) ;
#122284=CARTESIAN_POINT ( 'NONE',  ( 187.0052083336747444, -6.551208109652278289, 3.782341765624995134 ) ) ;
#122352=CARTESIAN_POINT ( 'NONE',  ( 186.9635416670080303, -4.367472073101520635, 7.564683531249999149 ) ) ;
#122376=VECTOR ( 'NONE', #29155, 1000.000000000000000 ) ;
#122384=CARTESIAN_POINT ( 'NONE',  ( 186.9062500006828316, -8.891194145520236347, -1.633285867636356299E-15 ) ) ;
#122520=CARTESIAN_POINT ( 'NONE',  ( 184.1510416670080588, 4.367472073101518859, -7.564683531249999149 ) ) ;
#122549=CARTESIAN_POINT ( 'NONE',  ( 184.2812500006828031, 0.000000000000000000, 7.700000000000000178 ) ) ;
#122582=CARTESIAN_POINT ( 'NONE',  ( 185.0729166673495172, 4.445597072760072876, -7.700000000000080114 ) ) ;
#122603=VERTEX_POINT ( 'NONE', #110841 ) ;
#122629=CARTESIAN_POINT ( 'NONE',  ( 184.0052083336747160, -6.551208109652278289, 3.782341765624995134 ) ) ;
#122685=DIRECTION ( 'NONE',  ( 1.000000000000000000, 0.000000000000000000, 0.000000000000000000 ) ) ;
#122720=DIRECTION ( 'NONE',  ( 0.000000000000000000, 0.000000000000000000, 1.000000000000000000 ) ) ;
#122768=VECTOR ( 'NONE', #34609, 1000.000000000000000 ) ;
#122809=DIRECTION ( 'NONE',  ( 1.000000000000000000, 0.000000000000000000, 0.000000000000000000 ) ) ;
#122823=( BOUNDED_CURVE ( )  B_SPLINE_CURVE ( 2, ( #104650, #112565, #33999, #122384, #124954, #54278, #114480 ),
 .UNSPECIFIED., .F., .F. ) 
 B_SPLINE_CURVE_WITH_KNOTS ( ( 3, 2, 2, 3 ),
 ( 0.07142857142857149400, 0.09523809523809532995, 0.1190476190476191520, 0.1428571428571429880 ),
 .UNSPECIFIED. ) 
 CURVE ( )  GEOMETRIC_REPRESENTATION_ITEM ( )  RATIONAL_B_SPLINE_CURVE ( ( 0.9999999999999996669, 0.8660254037844390407, 1.000000000000000000, 0.8660254037844387076, 1.000000000000000000, 0.8660254037844379305, 1.000000000000000666 ) ) 
 REPRESENTATION_ITEM ( '' )  );
#122877=CARTESIAN_POINT ( 'NONE',  ( 185.7395833340161460, 4.445597072760117285, 7.699999999999999289 ) ) ;
#122925=CARTESIAN_POINT ( 'NONE',  ( 184.2343750003414016, 8.734944146203032389, 5.348610694689227483E-16 ) ) ;
#122989=CARTESIAN_POINT ( 'NONE',  ( 187.4218750003414016, 0.000000000000000000, 7.564683531250000925 ) ) ;
#123018=CARTESIAN_POINT ( 'NONE',  ( 185.5312500006828031, 9.429780353434619030E-16, -7.700000000000000178 ) ) ;
#123042=LINE ( 'NONE', #41910, #6793 ) ;
#123166=CARTESIAN_POINT ( 'NONE',  ( 184.1093750003413732, 9.264065473108010111E-16, -7.564683531250000925 ) ) ;
#123188=ORIENTED_EDGE ( 'NONE', *, *, #76033, .F. ) ;
#123271=CARTESIAN_POINT ( 'NONE',  ( 186.9583333333333428, 4.445597072760117285, 7.699999999999999289 ) ) ;
#123501=CARTESIAN_POINT ( 'NONE',  ( 186.5729166673494603, 4.445597072760120838, -7.699999999999998401 ) ) ;
#123529=CARTESIAN_POINT ( 'NONE',  ( 187.5000000000000000, 0.000000000000000000, 0.000000000000000000 ) ) ;
#123536=DIRECTION ( 'NONE',  ( 0.000000000000000000, 0.000000000000000000, 1.000000000000000000 ) ) ;
#123542=CARTESIAN_POINT ( 'NONE',  ( 186.7552083336747444, 6.551208109652275624, -3.782341765624998686 ) ) ;
#123557=EDGE_CURVE ( 'NONE', #16283, #99145, #31084, .T. ) ;
#123595=LINE ( 'NONE', #33314, #122768 ) ;
#123663=CARTESIAN_POINT ( 'NONE',  ( 103.6810955943362558, 7.274704100468963652, -2.539691767268741351 ) ) ;
#123670=DIRECTION ( 'NONE',  ( 0.4999999999999471534, 0.000000000000000000, -0.8660254037844692387 ) ) ;
#123720=EDGE_CURVE ( 'NONE', #16557, #111056, #13232, .T. ) ;
#123904=CARTESIAN_POINT ( 'NONE',  ( 185.7135416670080588, 4.367472073101518859, -7.564683531249999149 ) ) ;
#123952=CYLINDRICAL_SURFACE ( 'NONE', #32577, 7.700000000000000178 ) ;
#124050=DIRECTION ( 'NONE',  ( 0.000000000000000000, -1.000000000000000000, 0.000000000000000000 ) ) ;
#124062=CARTESIAN_POINT ( 'NONE',  ( 183.7812500006828031, 0.000000000000000000, 7.700000000000000178 ) ) ;
#124153=CARTESIAN_POINT ( 'NONE',  ( 186.0729166673494319, 4.445597072760120838, -7.699999999999998401 ) ) ;
#124181=B_SPLINE_CURVE_WITH_KNOTS ( 'NONE', 3,
 ( #9226, #49173, #50433, #70720, #119175, #29514, #69419, #59646, #99551, #80553, #9871, #120465, #39984, #30820, #110641, #100805, #91648, #12431, #72024, #1967, #51735, #22288, #81818, #73289, #34019, #33394, #43858, #113208, #102743, #123663, #113872, #103409, #23546, #74587, #43216, #41918, #34683, #24203, #102120, #44476, #53657 ),
 .UNSPECIFIED., .F., .F.,
 ( 4, 2, 2, 2, 2, 2, 2, 2, 2, 2, 2, 1, 2, 2, 2, 2, 2, 2, 2, 2, 4 ),
 ( 0.01611678554250517079, 0.01712107061916237974, 0.01762321315749096687, 0.01812535569581955053, 0.01912964077247668315, 0.02013392584913381925, 0.02113821092579095187, 0.02164035346411951818, 0.02214249600244808103, 0.02314678107910519977, 0.02364892361743375915, 0.02415106615576231505, 0.02465320869409087443, 0.02515535123241943033, 0.02615963630907655602, 0.02716392138573368170, 0.02816820646239080739, 0.02917249153904793307, 0.03017677661570505876, 0.03118106169236218098, 0.03218534676901930319 ),
 .UNSPECIFIED. ) ;
#124217=ADVANCED_FACE ( 'NONE', ( #86004 ), #110591, .F. ) ;
#124248=CYLINDRICAL_SURFACE ( 'NONE', #96784, 3.000000000000000444 ) ;
#124279=CARTESIAN_POINT ( 'NONE',  ( 186.7552083336747444, 6.551208109652275624, -3.782341765624998686 ) ) ;
#124363=( BOUNDED_CURVE ( )  B_SPLINE_CURVE ( 2, ( #6784, #24531, #75544, #104375, #23898, #54617, #63818 ),
 .UNSPECIFIED., .F., .T. ) 
 B_SPLINE_CURVE_WITH_KNOTS ( ( 3, 2, 2, 3 ),
 ( 0.7857142857142862535, 0.8095238095238102005, 0.8333333333333340365, 0.8571428571428578724 ),
 .UNSPECIFIED. ) 
 CURVE ( )  GEOMETRIC_REPRESENTATION_ITEM ( )  RATIONAL_B_SPLINE_CURVE ( ( 0.9999999999999968914, 0.8660254037844418162, 1.000000000000000000, 0.8660254037844387076, 1.000000000000000000, 0.8660254037844343777, 1.000000000000004441 ) ) 
 REPRESENTATION_ITEM ( '' )  );
#124525=( NAMED_UNIT ( * ) PLANE_ANGLE_UNIT ( ) SI_UNIT ( $, .RADIAN. ) );
#124544=AXIS2_PLACEMENT_3D ( 'NONE', #57171, #127847, #125276 ) ;
#124552=DIRECTION ( 'NONE',  ( 1.000000000000000000, 0.000000000000000000, 0.000000000000000000 ) ) ;
#124567=CARTESIAN_POINT ( 'NONE',  ( 184.9635416670080872, -4.367472073101519747, 7.564683531249999149 ) ) ;
#124787=CARTESIAN_POINT ( 'NONE',  ( 186.8750000000000000, 8.891194145520236347, 5.444286225454521982E-16 ) ) ;
#124791=FACE_OUTER_BOUND ( 'NONE', #84488, .T. ) ;
#124809=CARTESIAN_POINT ( 'NONE',  ( 184.1562500006828316, 8.891194145520236347, 5.444286225454521982E-16 ) ) ;
#124820=FACE_OUTER_BOUND ( 'NONE', #120379, .T. ) ;
#124821=DIRECTION ( 'NONE',  ( 1.000000000000000000, 0.000000000000000000, 0.000000000000000000 ) ) ;
#124847=CARTESIAN_POINT ( 'NONE',  ( 179.5000000000000000, 0.000000000000000000, -6.000000000000000000 ) ) ;
#124954=CARTESIAN_POINT ( 'NONE',  ( 186.8645833340161175, -6.668395609140180369, 3.849999999999994760 ) ) ;
#124969=CARTESIAN_POINT ( 'NONE',  ( 109.3256943381949071, 5.995380816577922545, -4.832476092287897096 ) ) ;
#125204=CARTESIAN_POINT ( 'NONE',  ( 187.5000000000000000, 0.000000000000000000, 7.700000000000000178 ) ) ;
#125237=VERTEX_POINT ( 'NONE', #104170 ) ;
#125276=DIRECTION ( 'NONE',  ( 0.000000000000000000, 0.000000000000000000, -1.000000000000000000 ) ) ;
#125313=EDGE_CURVE ( 'NONE', #94142, #99145, #64872, .T. ) ;
#125351=EDGE_CURVE ( 'NONE', #61737, #2171, #67429, .T. ) ;
#125372=ORIENTED_EDGE ( 'NONE', *, *, #20926, .F. ) ;
#125392=EDGE_CURVE ( 'NONE', #80186, #128041, #121289, .T. ) ;
#125406=DIRECTION ( 'NONE',  ( 0.000000000000000000, 1.000000000000000000, -1.846105847067148761E-16 ) ) ;
#125444=CARTESIAN_POINT ( 'NONE',  ( 184.5312500006828031, 9.429780353434619030E-16, -7.700000000000000178 ) ) ;
#125486=CARTESIAN_POINT ( 'NONE',  ( 184.8385416670080872, 6.551208109652274736, 3.782341765625001351 ) ) ;
#125549=CARTESIAN_POINT ( 'NONE',  ( 185.1302083336747728, -4.367472073101514418, -7.564683531250002702 ) ) ;
#125709=APPLICATION_CONTEXT ( 'automotive_design' ) ;
#125832=CARTESIAN_POINT ( 'NONE',  ( 185.2916666666666572, 4.445597072760120838, -7.699999999999998401 ) ) ;
#125955=CARTESIAN_POINT ( 'NONE',  ( 186.1666666666666856, -6.668395609140176816, -3.850000000000003642 ) ) ;
#126049=DIRECTION ( 'NONE',  ( -0.000000000000000000, 1.000000000000000000, 1.846105847067148022E-16 ) ) ;
#126079=CARTESIAN_POINT ( 'NONE',  ( 186.6510416670080303, 4.367472073101518859, -7.564683531249999149 ) ) ;
#126100=DIRECTION ( 'NONE',  ( 1.000000000000000000, 0.000000000000000000, 0.000000000000000000 ) ) ;
#126205=CARTESIAN_POINT ( 'NONE',  ( 186.2968750003414584, 8.734944146203032389, 5.348610694689227483E-16 ) ) ;
#126217=EDGE_CURVE ( 'NONE', #51195, #65955, #37070, .T. ) ;
#126220=CARTESIAN_POINT ( 'NONE',  ( 129.5000000000000000, 0.6250000000000000000, 7.634788798650556707 ) ) ;
#126257=( BOUNDED_CURVE ( )  B_SPLINE_CURVE ( 2, ( #73260, #50394, #120433, #111904, #23508, #63447, #644 ),
 .UNSPECIFIED., .F., .F. ) 
 B_SPLINE_CURVE_WITH_KNOTS ( ( 3, 2, 2, 3 ),
 ( 0.1428571428571429880, 0.1666666666666668239, 0.1904761904761906322, 0.2142857142857144681 ),
 .UNSPECIFIED. ) 
 CURVE ( )  GEOMETRIC_REPRESENTATION_ITEM ( )  RATIONAL_B_SPLINE_CURVE ( ( 0.9999999999999992228, 0.8660254037844394848, 1.000000000000000000, 0.8660254037844387076, 1.000000000000000000, 0.8660254037844375974, 1.000000000000001110 ) ) 
 REPRESENTATION_ITEM ( '' )  );
#126401=VERTEX_POINT ( 'NONE', #43361 ) ;
#126496=CARTESIAN_POINT ( 'NONE',  ( 184.8333333333333144, 6.668395609140177704, -3.849999999999998312 ) ) ;
#126584=EDGE_CURVE ( 'NONE', #43268, #33034, #35467, .T. ) ;
#126626=CARTESIAN_POINT ( 'NONE',  ( 108.0000000000000142, 7.119691004531021328, -5.000000000000004441 ) ) ;
#126703=EDGE_CURVE ( 'NONE', #85963, #121068, #117865, .T. ) ;
#126724=ORIENTED_EDGE ( 'NONE', *, *, #43516, .F. ) ;
#126744=CARTESIAN_POINT ( 'NONE',  ( 185.0312500006828031, 9.429780353434619030E-16, -7.700000000000000178 ) ) ;
#126786=CARTESIAN_POINT ( 'NONE',  ( 183.9218750003414016, 0.000000000000000000, 7.564683531250000925 ) ) ;
#126795=EDGE_CURVE ( 'NONE', #103176, #31133, #62830, .T. ) ;
#126810=CARTESIAN_POINT ( 'NONE',  ( 185.5000000000000000, 0.000000000000000000, 7.700000000000000178 ) ) ;
#126857=CARTESIAN_POINT ( 'NONE',  ( 184.0885416670080872, -6.551208109652273848, -3.782341765625003571 ) ) ;
#126931=CARTESIAN_POINT ( 'NONE',  ( 187.0000000000000000, 0.000000000000000000, 7.700000000000000178 ) ) ;
#127086=( LENGTH_UNIT ( ) NAMED_UNIT ( * ) SI_UNIT ( .MILLI., .METRE. ) );
#127149=CARTESIAN_POINT ( 'NONE',  ( 184.9166666666666856, 6.668395609140176816, 3.850000000000000977 ) ) ;
#127154=VECTOR ( 'NONE', #21642, 1000.000000000000000 ) ;
#127292=CIRCLE ( 'NONE', #121020, 8.699999999999999289 ) ;
#127301=CARTESIAN_POINT ( 'NONE',  ( 129.5000000000000000, -1.500000000000000000, -2.598076211353316900 ) ) ;
#127374=ORIENTED_EDGE ( 'NONE', *, *, #123720, .F. ) ;
#127388=CARTESIAN_POINT ( 'NONE',  ( 186.3177083336747160, 4.367472073101515306, 7.564683531250000925 ) ) ;
#127473=EDGE_CURVE ( 'NONE', #86071, #101564, #66527, .T. ) ;
#127501=CARTESIAN_POINT ( 'NONE',  ( 185.8385416670080872, 6.551208109652274736, 3.782341765625001351 ) ) ;
#127522=CARTESIAN_POINT ( 'NONE',  ( 187.5000000000000000, 0.000000000000000000, 7.700000000000000178 ) ) ;
#127544=CARTESIAN_POINT ( 'NONE',  ( 112.7275879503070115, 7.525284458381443109, -1.660393549188459383 ) ) ;
#127546=DIRECTION ( 'NONE',  ( 1.000000000000000000, 0.000000000000000000, 0.000000000000000000 ) ) ;
#127576=DIRECTION ( 'NONE',  ( 1.000000000000000000, 0.000000000000000000, 0.000000000000000000 ) ) ;
#127582=CARTESIAN_POINT ( 'NONE',  ( 186.9843750003414300, -8.734944146203032389, -1.604583208406768146E-15 ) ) ;
#127679=VERTEX_POINT ( 'NONE', #354 ) ;
#127775=CARTESIAN_POINT ( 'NONE',  ( 185.2500000000000000, 9.429780353434619030E-16, -7.700000000000000178 ) ) ;
#127847=DIRECTION ( 'NONE',  ( 1.000000000000000000, 0.000000000000000000, 0.000000000000000000 ) ) ;
#128025=CARTESIAN_POINT ( 'NONE',  ( 185.9010416670080303, -4.367472073101519747, 7.564683531249999149 ) ) ;
#128041=VERTEX_POINT ( 'NONE', #66493 ) ;
#128062=FACE_OUTER_BOUND ( 'NONE', #12714, .T. ) ;
#128098=CARTESIAN_POINT ( 'NONE',  ( 185.3333333333333144, 6.668395609140177704, -3.849999999999998312 ) ) ;
#128120=CIRCLE ( 'NONE', #98769, 3.000000000000000444 ) ;
#128144=DIRECTION ( 'NONE',  ( 1.000000000000000000, 0.000000000000000000, 0.000000000000000000 ) ) ;
#128165=ORIENTED_EDGE ( 'NONE', *, *, #3193, .F. ) ;
#128193=CARTESIAN_POINT ( 'NONE',  ( 109.6525664375320304, 6.077905868614581486, 4.730106526360415842 ) ) ;
#128200=DIRECTION ( 'NONE',  ( 0.000000000000000000, 0.000000000000000000, -1.000000000000000000 ) ) ;
#128242=CARTESIAN_POINT ( 'NONE',  ( 185.8593750003413732, 0.000000000000000000, 7.564683531250000925 ) ) ;
#128369=CARTESIAN_POINT ( 'NONE',  ( 179.5000000000000000, -1.375000000000000000, 7.634788798650553154 ) ) ;
#128449=CARTESIAN_POINT ( 'NONE',  ( 186.2083333333333144, -4.445597072760115509, -7.700000000000001954 ) ) ;
#128544=CARTESIAN_POINT ( 'NONE',  ( 185.2083333333333144, -4.445597072760163471, -7.699999999999919353 ) ) ;
#128563=ORIENTED_EDGE ( 'NONE', *, *, #97903, .T. ) ;
#128706=CARTESIAN_POINT ( 'NONE',  ( 184.8177083336747160, 4.367472073101515306, 7.564683531250000925 ) ) ;
#128722=VERTEX_POINT ( 'NONE', #118665 ) ;
#128795=EDGE_CURVE ( 'NONE', #110378, #117106, #75395, .T. ) ;
#128796=EDGE_LOOP ( 'NONE', ( #128563, #2347, #12991, #110244 ) ) ;
#128847=CARTESIAN_POINT ( 'NONE',  ( 179.5000000000000000, -0.6250000000000025535, -6.000000000000000888 ) ) ;
#128855=ORIENTED_EDGE ( 'NONE', *, *, #126795, .F. ) ;
#128861=CARTESIAN_POINT ( 'NONE',  ( 108.1697673669222581, 5.855766388782916110, 5.000000000000030198 ) ) ;
#128979=CARTESIAN_POINT ( 'NONE',  ( 127.5000000000000000, -1.500000000000000000, 2.598076211353316900 ) ) ;
#128993=CIRCLE ( 'NONE', #72545, 8.699999999999999289 ) ;
#129028=ORIENTED_EDGE ( 'NONE', *, *, #11308, .F. ) ;
#129039=CARTESIAN_POINT ( 'NONE',  ( 179.5000000000000000, 0.6250000000000000000, 7.634788798650556707 ) ) ;
#129145=CARTESIAN_POINT ( 'NONE',  ( 186.7343750003414016, 8.734944146203032389, 5.348610694689227483E-16 ) ) ;
#129197=CARTESIAN_POINT ( 'NONE',  ( 179.5000000000000000, -1.375000000000000000, 7.634788798650553154 ) ) ;
#129240=ADVANCED_FACE ( 'NONE', ( #63300 ), #44439, .F. ) ;
#129254=CARTESIAN_POINT ( 'NONE',  ( 186.8802083336747444, 4.367472073101515306, 7.564683531250000925 ) ) ;
#129506=CARTESIAN_POINT ( 'NONE',  ( 107.9999999999992895, 5.855766388783293586, 5.000000000000080824 ) ) ;
#129520=DIRECTION ( 'NONE',  ( -0.000000000000000000, 1.000000000000000000, 1.846105847067148022E-16 ) ) ;
#129524=ORIENTED_EDGE ( 'NONE', *, *, #73107, .F. ) ;
#129532=CARTESIAN_POINT ( 'NONE',  ( 185.7500000000000000, 9.429780353434619030E-16, -7.700000000000000178 ) ) ;
#129543=CARTESIAN_POINT ( 'NONE',  ( 186.7343750003414300, 8.734944146203032389, 5.348610694689227483E-16 ) ) ;
#129597=VERTEX_POINT ( 'NONE', #91171 ) ;
ENDSEC;
END-ISO-10303-21;
